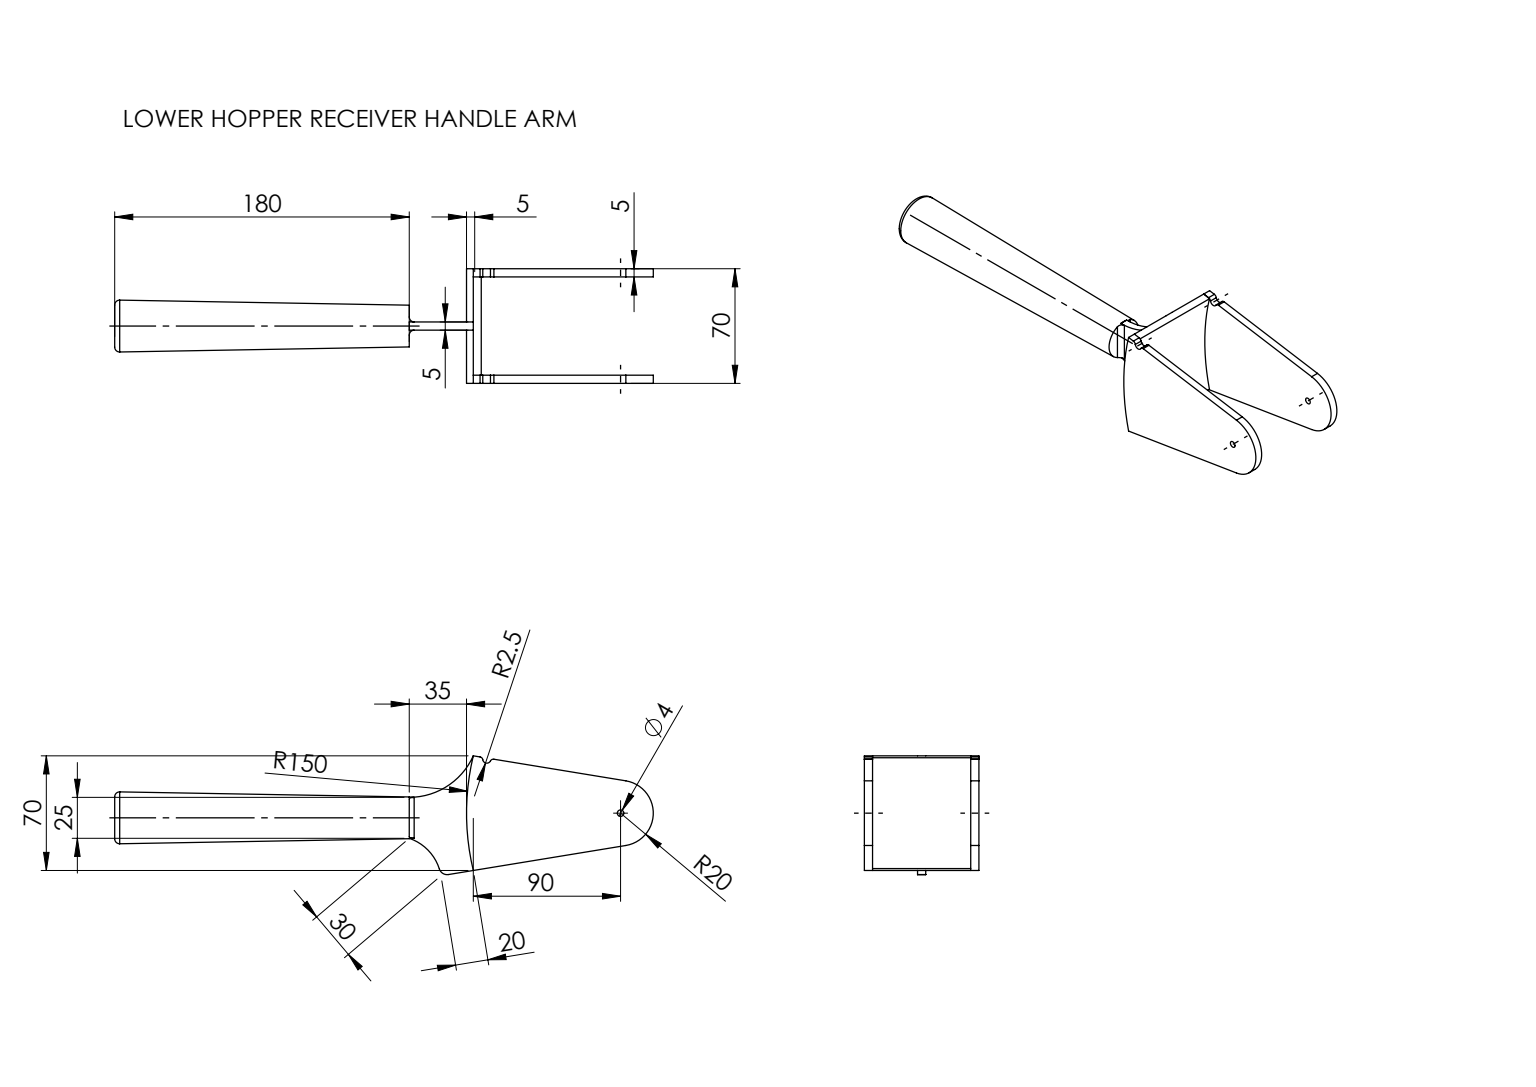
ISO-10303-21;
HEADER;
FILE_DESCRIPTION (('STEP AP214'),
    '1' );
FILE_NAME ('Lower Hopper Receiver Handle Arm.step',
    '2026-10-02T13:02:33',
    ( '' ),
    ( '' ),
    'SwSTEP 2.0',
    'SolidWorks 2026',
    '' );
FILE_SCHEMA (( 'AUTOMOTIVE_DESIGN' ));
ENDSEC;

DATA;
#29=LINE ( 'NONE', #5530, #5145 ) ;
#39=LINE ( 'NONE', #5829, #1016 ) ;
#44=VERTEX_POINT ( 'NONE', #12516 ) ;
#55=EDGE_CURVE ( 'NONE', #14250, #12234, #5712, .T. ) ;
#59=CIRCLE ( 'NONE', #13963, 20.00000000000001066 ) ;
#65=AXIS2_PLACEMENT_3D ( 'NONE', #12198, #9374, #18037 ) ;
#85=ADVANCED_FACE ( 'NONE', ( #5892 ), #18647, .T. ) ;
#86=CARTESIAN_POINT ( 'NONE',  ( -89.99999999999998579, -35.00000000000001421, 100.5765140304660861 ) ) ;
#96=CARTESIAN_POINT ( 'NONE',  ( -127.1404785156000941, 9.613695087247878135, -2.500000000000000000 ) ) ;
#99=CARTESIAN_POINT ( 'NONE',  ( -129.1404785418517918, 9.649298036820672664, 2.500000000000000000 ) ) ;
#111=CARTESIAN_POINT ( 'NONE',  ( 0.000000000000000000, 0.000000000000000000, 35.00000000000000000 ) ) ;
#116=DIRECTION ( 'NONE',  ( -0.9723968097209879646, 0.2333333333333338921, -0.000000000000000000 ) ) ;
#122=EDGE_LOOP ( 'NONE', ( #6243, #4264, #10759 ) ) ;
#125=ORIENTED_EDGE ( 'NONE', *, *, #6218, .F. ) ;
#126=CARTESIAN_POINT ( 'NONE',  ( -306.1404785418517918, -2.850701963179328668, 9.951701414186818625E-16 ) ) ;
#127=EDGE_CURVE ( 'NONE', #15127, #18093, #8457, .T. ) ;
#148=EDGE_CURVE ( 'NONE', #7107, #5722, #1632, .T. ) ;
#150=EDGE_CURVE ( 'NONE', #1792, #949, #14691, .T. ) ;
#190=CIRCLE ( 'NONE', #802, 42.89102435249441925 ) ;
#198=DIRECTION ( 'NONE',  ( 1.000000000000000000, 0.000000000000000000, -0.000000000000000000 ) ) ;
#215=EDGE_LOOP ( 'NONE', ( #10832, #6172, #11697, #10724 ) ) ;
#237=LINE ( 'NONE', #7306, #7511 ) ;
#245=CARTESIAN_POINT ( 'NONE',  ( -129.1404785418517918, 8.649298036820676217, 5.500000000000000000 ) ) ;
#246=CYLINDRICAL_SURFACE ( 'NONE', #528, 2.000000000000001776 ) ;
#266=FACE_OUTER_BOUND ( 'NONE', #3188, .T. ) ;
#273=EDGE_CURVE ( 'NONE', #17252, #3975, #18174, .T. ) ;
#286=AXIS2_PLACEMENT_3D ( 'NONE', #9882, #15657, #10154 ) ;
#290=ORIENTED_EDGE ( 'NONE', *, *, #11265, .T. ) ;
#294=VERTEX_POINT ( 'NONE', #7445 ) ;
#305=ORIENTED_EDGE ( 'NONE', *, *, #9387, .T. ) ;
#348=VECTOR ( 'NONE', #6882, 1000.000000000000000 ) ;
#381=ORIENTED_EDGE ( 'NONE', *, *, #387, .F. ) ;
#387=EDGE_CURVE ( 'NONE', #11399, #16710, #13584, .T. ) ;
#429=ORIENTED_EDGE ( 'NONE', *, *, #3774, .F. ) ;
#482=VERTEX_POINT ( 'NONE', #1195 ) ;
#514=CARTESIAN_POINT ( 'NONE',  ( -129.1404785418517918, -2.850701963179328668, 9.951701414186818625E-16 ) ) ;
#528=AXIS2_PLACEMENT_3D ( 'NONE', #2893, #8689, #14567 ) ;
#551=FILL_AREA_STYLE_COLOUR ( '', #12034 ) ;
#569=CIRCLE ( 'NONE', #2365, 150.0000000000000000 ) ;
#580=UNCERTAINTY_MEASURE_WITH_UNIT (LENGTH_MEASURE( 1.000000000000000082E-05 ), #14853, 'distance_accuracy_value', 'NONE');
#582=FACE_OUTER_BOUND ( 'NONE', #8107, .T. ) ;
#584=VERTEX_POINT ( 'NONE', #8328 ) ;
#610=VERTEX_POINT ( 'NONE', #13044 ) ;
#634=ADVANCED_FACE ( 'NONE', ( #824 ), #15404, .T. ) ;
#648=AXIS2_PLACEMENT_3D ( 'NONE', #10093, #14649, #17614 ) ;
#650=CARTESIAN_POINT ( 'NONE',  ( 55.85952145814821534, 6.938893903907228378E-15, -30.00000000000000000 ) ) ;
#651=DIRECTION ( 'NONE',  ( 0.000000000000000000, 0.000000000000000000, 1.000000000000000000 ) ) ;
#660=TOROIDAL_SURFACE ( 'NONE', #5229, 12.83663829214476060, 3.000000000000000000 ) ;
#668=EDGE_LOOP ( 'NONE', ( #10359, #125, #12635, #15355, #1976 ) ) ;
#669=EDGE_CURVE ( 'NONE', #3382, #9105, #9816, .T. ) ;
#678=CARTESIAN_POINT ( 'NONE',  ( -129.1404785418517918, -2.850701963179328668, 9.951701414186818625E-16 ) ) ;
#715=DIRECTION ( 'NONE',  ( 0.9868632313631133801, 0.1615579233078775490, 0.000000000000000000 ) ) ;
#716=DIRECTION ( 'NONE',  ( -2.735665993912342121E-16, -0.000000000000000000, -1.000000000000000000 ) ) ;
#733=EDGE_LOOP ( 'NONE', ( #1309, #17633, #9167, #16624 ) ) ;
#739=CARTESIAN_POINT ( 'NONE',  ( 3.231158466157545206, -19.73726462726228092, -35.00000000000000000 ) ) ;
#746=CARTESIAN_POINT ( 'NONE',  ( -306.0881213225399051, -2.850701963179326448, -15.83618137761393463 ) ) ;
#765=CARTESIAN_POINT ( 'NONE',  ( -128.8626752476364175, -14.87423233749613694, -4.224609204322598011 ) ) ;
#766=DIRECTION ( 'NONE',  ( -0.000000000000000000, -0.000000000000000000, -1.000000000000000000 ) ) ;
#768=CARTESIAN_POINT ( 'NONE',  ( -127.1354840320379225, 9.580137489138413898, -2.662644313562638754 ) ) ;
#769=DIRECTION ( 'NONE',  ( -0.000000000000000000, -0.000000000000000000, -1.000000000000000000 ) ) ;
#787=EDGE_CURVE ( 'NONE', #17205, #5608, #12280, .T. ) ;
#802=AXIS2_PLACEMENT_3D ( 'NONE', #11740, #14986, #10707 ) ;
#804=CARTESIAN_POINT ( 'NONE',  ( -126.1404785418517918, -15.29729532696464922, 2.500000000000000000 ) ) ;
#820=ORIENTED_EDGE ( 'NONE', *, *, #55, .F. ) ;
#822=COLOUR_RGB ( '', 0.09019608, 0.27058824, 0.51372549) ;
#824=FACE_OUTER_BOUND ( 'NONE', #12213, .T. ) ;
#846=DIRECTION ( 'NONE',  ( 0.000000000000000000, -1.000000000000000000, 0.000000000000000000 ) ) ;
#861=CARTESIAN_POINT ( 'NONE',  ( -129.1404785418517918, -15.35070196317932911, -2.500000000000000000 ) ) ;
#866=DIRECTION ( 'NONE',  ( 1.000000000000000000, -3.469446951953611033E-15, 0.000000000000000000 ) ) ;
#870=CARTESIAN_POINT ( 'NONE',  ( -77.72973689007648090, 30.96463005215034059, 30.00000000000002842 ) ) ;
#876=ORIENTED_EDGE ( 'NONE', *, *, #14228, .F. ) ;
#915=LINE ( 'NONE', #14158, #348 ) ;
#935=VECTOR ( 'NONE', #846, 1000.000000000000000 ) ;
#949=VERTEX_POINT ( 'NONE', #14168 ) ;
#970=CYLINDRICAL_SURFACE ( 'NONE', #18454, 42.89102435249441925 ) ;
#978=EDGE_CURVE ( 'NONE', #14250, #3442, #3727, .T. ) ;
#986=CARTESIAN_POINT ( 'NONE',  ( -129.1404785418517918, -2.850701963179328668, 9.951701414186818625E-16 ) ) ;
#1000=LINE ( 'NONE', #6771, #7871 ) ;
#1012=ADVANCED_FACE ( 'NONE', ( #3813 ), #9628, .F. ) ;
#1016=VECTOR ( 'NONE', #13635, 1000.000000000000000 ) ;
#1025=CYLINDRICAL_SURFACE ( 'NONE', #1765, 150.0000000000000000 ) ;
#1026=CARTESIAN_POINT ( 'NONE',  ( 0.000000000000000000, 0.000000000000000000, 35.00000000000000000 ) ) ;
#1037=ORIENTED_EDGE ( 'NONE', *, *, #6093, .T. ) ;
#1043=AXIS2_PLACEMENT_3D ( 'NONE', #16101, #1684, #10478 ) ;
#1070=CARTESIAN_POINT ( 'NONE',  ( -79.50968810220766159, 31.87664632526870889, -35.00000000000000000 ) ) ;
#1071=ADVANCED_FACE ( 'NONE', ( #5585 ), #1143, .F. ) ;
#1094=ORIENTED_EDGE ( 'NONE', *, *, #9224, .T. ) ;
#1121=CIRCLE ( 'NONE', #15923, 150.0000000000000000 ) ;
#1124=DIRECTION ( 'NONE',  ( -1.000000000000000000, 0.000000000000000000, 0.000000000000000000 ) ) ;
#1137=CARTESIAN_POINT ( 'NONE',  ( -80.37374032648909861, 30.90317544272717498, 35.00001199999999102 ) ) ;
#1143=CYLINDRICAL_SURFACE ( 'NONE', #11190, 145.0000000000000284 ) ;
#1150=B_SPLINE_CURVE_WITH_KNOTS ( 'NONE', 3,
 ( #99, #8902, #14865, #6255 ),
 .UNSPECIFIED., .F., .F.,
 ( 4, 4 ),
 ( 0.000000000000000000, 0.003000475340473869428 ),
 .UNSPECIFIED. ) ;
#1153=CARTESIAN_POINT ( 'NONE',  ( -128.4401431403265121, 9.376841461187488846, -3.563338245596201048 ) ) ;
#1161=CARTESIAN_POINT ( 'NONE',  ( -128.1404785157144204, 9.631497293019437578, -2.500000000000000000 ) ) ;
#1184=CARTESIAN_POINT ( 'NONE',  ( -90.00000000000000000, 34.99999999999999289, -2.499999999999974243 ) ) ;
#1195=CARTESIAN_POINT ( 'NONE',  ( -77.40662104346073136, 32.93835651487657401, -35.00000000000000000 ) ) ;
#1245=CARTESIAN_POINT ( 'NONE',  ( -110.7369027592740167, -34.07064978273316314, -2.500000000000000000 ) ) ;
#1247=LINE ( 'NONE', #7032, #4023 ) ;
#1255=DIRECTION ( 'NONE',  ( -2.735665993912342121E-16, -0.000000000000000000, -1.000000000000000000 ) ) ;
#1256=VECTOR ( 'NONE', #2851, 1000.000000000000000 ) ;
#1272=ORIENTED_EDGE ( 'NONE', *, *, #9509, .T. ) ;
#1274=CARTESIAN_POINT ( 'NONE',  ( -129.1404785418517918, 9.649298036820672664, 2.500000000000000000 ) ) ;
#1286=ORIENTED_EDGE ( 'NONE', *, *, #15705, .F. ) ;
#1287=DIRECTION ( 'NONE',  ( 0.000000000000000000, 0.000000000000000000, 1.000000000000000000 ) ) ;
#1309=ORIENTED_EDGE ( 'NONE', *, *, #1355, .F. ) ;
#1311=CYLINDRICAL_SURFACE ( 'NONE', #648, 2.000000000000001776 ) ;
#1312=VERTEX_POINT ( 'NONE', #13991 ) ;
#1325=EDGE_LOOP ( 'NONE', ( #11302, #17504, #9683, #6379 ) ) ;
#1341=FACE_OUTER_BOUND ( 'NONE', #6254, .T. ) ;
#1342=DIRECTION ( 'NONE',  ( 0.000000000000000000, 0.000000000000000000, 1.000000000000000000 ) ) ;
#1347=CARTESIAN_POINT ( 'NONE',  ( -90.00000000000000000, 34.99999999999999289, -30.00000000000000000 ) ) ;
#1355=EDGE_CURVE ( 'NONE', #13473, #12774, #14782, .T. ) ;
#1356=CYLINDRICAL_SURFACE ( 'NONE', #8842, 2.500000000000002220 ) ;
#1360=ORIENTED_EDGE ( 'NONE', *, *, #12905, .F. ) ;
#1363=CARTESIAN_POINT ( 'NONE',  ( -90.00000000000000000, 34.99999999999999289, -30.00000000000000000 ) ) ;
#1364=CARTESIAN_POINT ( 'NONE',  ( -126.1404785418517918, 6.938893903907228378E-15, 5.500000000000000000 ) ) ;
#1371=DIRECTION ( 'NONE',  ( 0.000000000000000000, 0.000000000000000000, 1.000000000000000000 ) ) ;
#1385=DIRECTION ( 'NONE',  ( 0.000000000000000000, 0.000000000000000000, -1.000000000000000000 ) ) ;
#1476=ORIENTED_EDGE ( 'NONE', *, *, #6473, .T. ) ;
#1483=DIRECTION ( 'NONE',  ( -0.000000000000000000, -0.000000000000000000, -1.000000000000000000 ) ) ;
#1485=AXIS2_PLACEMENT_3D ( 'NONE', #7363, #4399, #17328 ) ;
#1487=CARTESIAN_POINT ( 'NONE',  ( -126.1404785418517918, -15.29729532696464922, 2.500000000000000000 ) ) ;
#1494=EDGE_CURVE ( 'NONE', #13776, #10500, #13396, .T. ) ;
#1523=CYLINDRICAL_SURFACE ( 'NONE', #16034, 2.000000000000000000 ) ;
#1614=VERTEX_POINT ( 'NONE', #3435 ) ;
#1616=DIRECTION ( 'NONE',  ( 3.039628882124824168E-17, 0.000000000000000000, -1.000000000000000000 ) ) ;
#1623=DIRECTION ( 'NONE',  ( -1.000000000000000000, 0.000000000000000000, 0.000000000000000000 ) ) ;
#1627=ADVANCED_FACE ( 'NONE', ( #9323 ), #18078, .F. ) ;
#1628=ADVANCED_FACE ( 'NONE', ( #16839 ), #9613, .T. ) ;
#1632=LINE ( 'NONE', #7692, #9344 ) ;
#1656=CARTESIAN_POINT ( 'NONE',  ( -77.40662104346073136, 32.93835651487657401, 35.00000000000000000 ) ) ;
#1680=VERTEX_POINT ( 'NONE', #2865 ) ;
#1684=DIRECTION ( 'NONE',  ( 2.735665993912342121E-16, 0.000000000000000000, 1.000000000000000000 ) ) ;
#1685=ORIENTED_EDGE ( 'NONE', *, *, #10006, .F. ) ;
#1687=SURFACE_STYLE_USAGE ( .BOTH. , #11800 ) ;
#1707=DIRECTION ( 'NONE',  ( -0.000000000000000000, -0.000000000000000000, 1.000000000000000000 ) ) ;
#1718=ADVANCED_FACE ( 'NONE', ( #17513 ), #12778, .F. ) ;
#1726=CARTESIAN_POINT ( 'NONE',  ( -129.1404785418517918, -2.850701963179328668, 9.951701414186818625E-16 ) ) ;
#1727=VECTOR ( 'NONE', #15326, 1000.000000000000000 ) ;
#1733=EDGE_CURVE ( 'NONE', #18389, #16485, #12664, .T. ) ;
#1747=ORIENTED_EDGE ( 'NONE', *, *, #13227, .T. ) ;
#1761=EDGE_LOOP ( 'NONE', ( #6420, #11707, #14054, #2020 ) ) ;
#1765=AXIS2_PLACEMENT_3D ( 'NONE', #9732, #14062, #18386 ) ;
#1772=AXIS2_PLACEMENT_3D ( 'NONE', #111, #4368, #14237 ) ;
#1792=VERTEX_POINT ( 'NONE', #15900 ) ;
#1793=ADVANCED_FACE ( 'NONE', ( #4423 ), #6927, .F. ) ;
#1836=DIRECTION ( 'NONE',  ( -0.000000000000000000, -0.000000000000000000, -1.000000000000000000 ) ) ;
#1852=EDGE_CURVE ( 'NONE', #5489, #2351, #11341, .T. ) ;
#1857=SURFACE_SIDE_STYLE ('',( #13401 ) ) ;
#1860=FACE_OUTER_BOUND ( 'NONE', #5789, .T. ) ;
#1873=CARTESIAN_POINT ( 'NONE',  ( -129.1404785418517918, 8.649298036820674440, -5.500000000000000000 ) ) ;
#1875=DIRECTION ( 'NONE',  ( 1.000000000000000000, 0.000000000000000000, 0.000000000000000000 ) ) ;
#1876=ORIENTED_EDGE ( 'NONE', *, *, #18633, .T. ) ;
#1877=EDGE_CURVE ( 'NONE', #10500, #12364, #7467, .T. ) ;
#1900=DIRECTION ( 'NONE',  ( 1.000000000000000000, 0.000000000000000000, 0.000000000000000000 ) ) ;
#1925=DIRECTION ( 'NONE',  ( 1.000000000000000000, 0.000000000000000000, 0.000000000000000000 ) ) ;
#1942=CARTESIAN_POINT ( 'NONE',  ( 55.85952145814821534, 6.938893903907228378E-15, -2.500000000000000000 ) ) ;
#1943=CARTESIAN_POINT ( 'NONE',  ( -90.00000000000000000, 34.99999999999999289, 35.00000000000000000 ) ) ;
#1947=EDGE_CURVE ( 'NONE', #15938, #1312, #8966, .T. ) ;
#1961=CARTESIAN_POINT ( 'NONE',  ( -89.99999999999998579, -35.00000000000001421, 30.00000000000005329 ) ) ;
#1962=CYLINDRICAL_SURFACE ( 'NONE', #4186, 2.500000000000002220 ) ;
#1965=CARTESIAN_POINT ( 'NONE',  ( -90.00000000000000000, 34.99999999999999289, 35.00000000000000000 ) ) ;
#1975=EDGE_CURVE ( 'NONE', #10686, #18371, #915, .T. ) ;
#1976=ORIENTED_EDGE ( 'NONE', *, *, #16677, .F. ) ;
#1978=DIRECTION ( 'NONE',  ( 1.000000000000000000, 0.000000000000000000, 0.000000000000000000 ) ) ;
#1994=CIRCLE ( 'NONE', #13775, 150.0000000000000000 ) ;
#2011=ORIENTED_EDGE ( 'NONE', *, *, #15762, .T. ) ;
#2020=ORIENTED_EDGE ( 'NONE', *, *, #6851, .F. ) ;
#2038=DIRECTION ( 'NONE',  ( 0.000000000000000000, 0.000000000000000000, 1.000000000000000000 ) ) ;
#2054=CARTESIAN_POINT ( 'NONE',  ( -306.0881213225399051, -2.850701963179328668, 9.951701414186818625E-16 ) ) ;
#2056=AXIS2_PLACEMENT_3D ( 'NONE', #9834, #14191, #14294 ) ;
#2057=DIRECTION ( 'NONE',  ( -1.000000000000000000, 0.000000000000000000, 0.000000000000000000 ) ) ;
#2077=DIRECTION ( 'NONE',  ( 0.000000000000000000, 0.000000000000000000, -1.000000000000000000 ) ) ;
#2083=CARTESIAN_POINT ( 'NONE',  ( -90.00000000000000000, 34.99999999999999289, 35.00000000000000000 ) ) ;
#2084=DIRECTION ( 'NONE',  ( 1.000000000000000000, 0.000000000000000000, 0.000000000000000000 ) ) ;
#2105=CIRCLE ( 'NONE', #2707, 150.0000000000000000 ) ;
#2123=CARTESIAN_POINT ( 'NONE',  ( -86.18478963674542115, 32.34879426031891114, 30.00000000000002842 ) ) ;
#2133=VECTOR ( 'NONE', #18684, 1000.000000000000114 ) ;
#2146=CARTESIAN_POINT ( 'NONE',  ( 0.000000000000000000, 0.000000000000000000, 35.00000000000000000 ) ) ;
#2154=DIRECTION ( 'NONE',  ( -0.1615579233078772992, -0.9868632313631134911, 0.000000000000000000 ) ) ;
#2158=AXIS2_PLACEMENT_3D ( 'NONE', #7119, #12950, #4341 ) ;
#2176=ORIENTED_EDGE ( 'NONE', *, *, #11265, .F. ) ;
#2197=ORIENTED_EDGE ( 'NONE', *, *, #2667, .T. ) ;
#2202=DIRECTION ( 'NONE',  ( -0.000000000000000000, -0.000000000000000000, -1.000000000000000000 ) ) ;
#2208=ADVANCED_FACE ( 'NONE', ( #8277 ), #7046, .T. ) ;
#2216=ORIENTED_EDGE ( 'NONE', *, *, #5344, .F. ) ;
#2225=AXIS2_PLACEMENT_3D ( 'NONE', #3368, #16274, #10389 ) ;
#2248=CARTESIAN_POINT ( 'NONE',  ( -84.20837060243641758, 32.64545563739221024, 35.00000599999999906 ) ) ;
#2258=EDGE_LOOP ( 'NONE', ( #12744, #14922, #1094, #12317 ) ) ;
#2263=CIRCLE ( 'NONE', #18053, 2.000000000000001776 ) ;
#2264=DIRECTION ( 'NONE',  ( -1.000000000000000000, 0.000000000000000000, 0.000000000000000000 ) ) ;
#2287=AXIS2_PLACEMENT_3D ( 'NONE', #14317, #1342, #7124 ) ;
#2294=ORIENTED_EDGE ( 'NONE', *, *, #4880, .F. ) ;
#2301=CARTESIAN_POINT ( 'NONE',  ( -127.1354840320379225, -15.28154141549707035, 2.662644313562638310 ) ) ;
#2311=FACE_OUTER_BOUND ( 'NONE', #5865, .T. ) ;
#2314=DIRECTION ( 'NONE',  ( 0.000000000000000000, 1.000000000000000000, 1.224646799147353207E-16 ) ) ;
#2316=EDGE_LOOP ( 'NONE', ( #14529, #15736, #9747, #13850 ) ) ;
#2351=VERTEX_POINT ( 'NONE', #5911 ) ;
#2365=AXIS2_PLACEMENT_3D ( 'NONE', #3427, #17888, #6406 ) ;
#2371=CIRCLE ( 'NONE', #13861, 2.000000000000001776 ) ;
#2390=VERTEX_POINT ( 'NONE', #11928 ) ;
#2405=CARTESIAN_POINT ( 'NONE',  ( 55.85952145814821534, 6.938893903907228378E-15, 35.00000000000000000 ) ) ;
#2412=LINE ( 'NONE', #8380, #9979 ) ;
#2421=CARTESIAN_POINT ( 'NONE',  ( -84.20837060243641758, 32.64545563739221024, 35.00000599999999906 ) ) ;
#2449=CARTESIAN_POINT ( 'NONE',  ( -83.32982269052723723, 31.07393428812022051, 35.00001200000000523 ) ) ;
#2470=CARTESIAN_POINT ( 'NONE',  ( -126.5450966053943631, 9.599007176297428501, -2.520603730400377440 ) ) ;
#2471=DIRECTION ( 'NONE',  ( 0.000000000000000000, 0.000000000000000000, -1.000000000000000000 ) ) ;
#2477=CARTESIAN_POINT ( 'NONE',  ( -89.99999999999998579, -35.00000000000001421, 2.500000000000030198 ) ) ;
#2478=ORIENTED_EDGE ( 'NONE', *, *, #13227, .F. ) ;
#2492=AXIS2_PLACEMENT_3D ( 'NONE', #2054, #6442, #651 ) ;
#2502=EDGE_LOOP ( 'NONE', ( #15673, #8880, #4795, #16546, #6404 ) ) ;
#2514=FACE_BOUND ( 'NONE', #2700, .T. ) ;
#2531=SHAPE_REPRESENTATION_RELATIONSHIP ( 'NONE' , 'NONE' ,  #17876, #16831 ) ;
#2554=CARTESIAN_POINT ( 'NONE',  ( 55.85952145814821534, 6.938893903907228378E-15, 35.00000000000000000 ) ) ;
#2561=VERTEX_POINT ( 'NONE', #9480 ) ;
#2577=FACE_OUTER_BOUND ( 'NONE', #5940, .T. ) ;
#2578=DIRECTION ( 'NONE',  ( -0.9868632313631133801, 0.1615579233078772436, -0.000000000000000000 ) ) ;
#2606=EDGE_LOOP ( 'NONE', ( #4453, #290, #8768, #8101, #18259, #11902, #6738, #11595, #18767 ) ) ;
#2608=AXIS2_PLACEMENT_3D ( 'NONE', #4351, #18716, #16004 ) ;
#2616=VECTOR ( 'NONE', #2844, 1000.000000000000000 ) ;
#2622=DIRECTION ( 'NONE',  ( -1.000000000000000000, 0.000000000000000000, 0.000000000000000000 ) ) ;
#2624=ORIENTED_EDGE ( 'NONE', *, *, #1733, .F. ) ;
#2637=DIRECTION ( 'NONE',  ( -0.000000000000000000, -0.000000000000000000, -1.000000000000000000 ) ) ;
#2667=EDGE_CURVE ( 'NONE', #12027, #13473, #9158, .T. ) ;
#2671=DIRECTION ( 'NONE',  ( 0.000000000000000000, -1.000000000000000000, 0.000000000000000000 ) ) ;
#2674=ORIENTED_EDGE ( 'NONE', *, *, #14267, .F. ) ;
#2688=VECTOR ( 'NONE', #18062, 1000.000000000000000 ) ;
#2700=EDGE_LOOP ( 'NONE', ( #3536, #4135 ) ) ;
#2707=AXIS2_PLACEMENT_3D ( 'NONE', #1942, #12050, #17710 ) ;
#2713=CARTESIAN_POINT ( 'NONE',  ( -128.1677737538112751, 9.451028958170518024, 3.279750847804448366 ) ) ;
#2726=LINE ( 'NONE', #4126, #10310 ) ;
#2741=CARTESIAN_POINT ( 'NONE',  ( -85.86167379012967160, 34.32252072304513746, 35.00000000000000000 ) ) ;
#2775=ORIENTED_EDGE ( 'NONE', *, *, #6196, .F. ) ;
#2780=EDGE_CURVE ( 'NONE', #13776, #2561, #17653, .T. ) ;
#2842=ORIENTED_EDGE ( 'NONE', *, *, #15504, .F. ) ;
#2844=DIRECTION ( 'NONE',  ( -0.000000000000000000, -0.000000000000000000, -1.000000000000000000 ) ) ;
#2851=DIRECTION ( 'NONE',  ( -0.000000000000000000, -0.000000000000000000, -1.000000000000000000 ) ) ;
#2861=AXIS2_PLACEMENT_3D ( 'NONE', #15696, #2622, #10781 ) ;
#2865=CARTESIAN_POINT ( 'NONE',  ( -129.1404785418517918, -2.850701963179326892, -12.74754878398196389 ) ) ;
#2870=EDGE_CURVE ( 'NONE', #610, #12140, #10520, .T. ) ;
#2871=CARTESIAN_POINT ( 'NONE',  ( -129.1404785418517918, 9.649298036820672664, 2.500000000000000000 ) ) ;
#2883=CARTESIAN_POINT ( 'NONE',  ( -128.0167453206627783, 9.481696373754449070, 3.150553392547042364 ) ) ;
#2890=DIRECTION ( 'NONE',  ( 0.9868632313631133801, 0.1615579233078773547, -0.000000000000000000 ) ) ;
#2893=CARTESIAN_POINT ( 'NONE',  ( -86.18478963674542115, 32.34879426031891114, -35.00000000000000000 ) ) ;
#2895=CARTESIAN_POINT ( 'NONE',  ( -81.73462711737164454, 33.01666666666666572, -30.00000000000000355 ) ) ;
#2908=DIRECTION ( 'NONE',  ( -0.9868632313631133801, -0.1615579233078775490, 0.000000000000000000 ) ) ;
#2924=CIRCLE ( 'NONE', #15335, 29.12282187559191016 ) ;
#2941=FACE_OUTER_BOUND ( 'NONE', #733, .T. ) ;
#2951=CARTESIAN_POINT ( 'NONE',  ( -309.1404785418517918, -2.850701963179328668, 12.83663829214476237 ) ) ;
#2979=CARTESIAN_POINT ( 'NONE',  ( -84.20693962813486166, 32.64562644091790844, -35.00000000000000000 ) ) ;
#2998=EDGE_CURVE ( 'NONE', #7107, #13776, #10226, .T. ) ;
#3001=AXIS2_PLACEMENT_3D ( 'NONE', #3771, #13725, #6472 ) ;
#3023=ORIENTED_EDGE ( 'NONE', *, *, #787, .T. ) ;
#3027=ORIENTED_EDGE ( 'NONE', *, *, #1494, .F. ) ;
#3034=EDGE_LOOP ( 'NONE', ( #16222, #15224, #6139, #16013 ) ) ;
#3036=CARTESIAN_POINT ( 'NONE',  ( -129.1404785418517918, -14.35070196317933267, -5.500000000000000000 ) ) ;
#3044=DIRECTION ( 'NONE',  ( 1.000000000000000000, 0.000000000000000000, 0.000000000000000000 ) ) ;
#3046=FACE_OUTER_BOUND ( 'NONE', #2606, .T. ) ;
#3074=EDGE_LOOP ( 'NONE', ( #6524, #10962, #2478, #2775 ) ) ;
#3095=ORIENTED_EDGE ( 'NONE', *, *, #387, .T. ) ;
#3105=ADVANCED_FACE ( 'NONE', ( #16971 ), #17062, .F. ) ;
#3108=LINE ( 'NONE', #8899, #16953 ) ;
#3118=FACE_OUTER_BOUND ( 'NONE', #4884, .T. ) ;
#3160=DIRECTION ( 'NONE',  ( -0.1615579233078772992, -0.9868632313631134911, 0.000000000000000000 ) ) ;
#3163=PRESENTATION_STYLE_ASSIGNMENT (( #9236 ) ) ;
#3188=EDGE_LOOP ( 'NONE', ( #15172, #10918, #18610 ) ) ;
#3201=EDGE_CURVE ( 'NONE', #9794, #12027, #14443, .T. ) ;
#3213=MECHANICAL_DESIGN_GEOMETRIC_PRESENTATION_REPRESENTATION('',(#11387),#8064);
#3231=AXIS2_PLACEMENT_3D ( 'NONE', #15088, #4857, #16443 ) ;
#3243=ADVANCED_FACE ( 'NONE', ( #13217 ), #246, .T. ) ;
#3268=CLOSED_SHELL ( 'NONE', ( #9951, #4039, #1012, #1071, #1793, #1628, #5538, #10881, #3871, #14129, #18595, #12794, #85, #10346, #8273, #12172, #5357, #1718, #11643, #9411, #18632, #634, #13985, #3105, #4856, #13649, #18487, #1627, #18382, #14420, #13554, #13698, #12325, #5455, #11741, #8566, #11712, #11441, #2208, #7666, #18748, #3243, #13478, #7173, #7750, #17276, #15621 ) ) ;
#3272=CARTESIAN_POINT ( 'NONE',  ( -89.14047854185180597, 6.938893903907228378E-15, 100.5765140304660861 ) ) ;
#3304=CARTESIAN_POINT ( 'NONE',  ( -89.99999999999998579, -35.00000000000001421, 2.500000000000000000 ) ) ;
#3322=AXIS2_PLACEMENT_3D ( 'NONE', #7981, #15189, #10802 ) ;
#3330=CIRCLE ( 'NONE', #11804, 2.500000000000002220 ) ;
#3355=CARTESIAN_POINT ( 'NONE',  ( -86.18478963674542115, 32.34879426031891114, -30.00000000000000355 ) ) ;
#3357=AXIS2_PLACEMENT_3D ( 'NONE', #8174, #14036, #12600 ) ;
#3368=CARTESIAN_POINT ( 'NONE',  ( -90.00000000000000000, 34.99999999999999289, 100.5765140304660861 ) ) ;
#3382=VERTEX_POINT ( 'NONE', #9309 ) ;
#3389=LINE ( 'NONE', #12291, #6432 ) ;
#3391=CARTESIAN_POINT ( 'NONE',  ( -129.0554062880559343, -14.67359210495141575, -4.766626691765363688 ) ) ;
#3396=VERTEX_POINT ( 'NONE', #3424 ) ;
#3406=ORIENTED_EDGE ( 'NONE', *, *, #978, .F. ) ;
#3416=EDGE_CURVE ( 'NONE', #14596, #18395, #11106, .T. ) ;
#3420=CARTESIAN_POINT ( 'NONE',  ( -89.99999999999998579, -35.00000000000001421, 30.00000000000002487 ) ) ;
#3424=CARTESIAN_POINT ( 'NONE',  ( -79.50968810220766159, 31.87664632526870889, 30.00000000000002842 ) ) ;
#3427=CARTESIAN_POINT ( 'NONE',  ( 55.85952145814821534, 6.938893903907228378E-15, 2.500000000000000000 ) ) ;
#3435=CARTESIAN_POINT ( 'NONE',  ( -79.50968810220766159, 31.87664632526870889, -35.00000000000000000 ) ) ;
#3442=VERTEX_POINT ( 'NONE', #6944 ) ;
#3445=ORIENTED_EDGE ( 'NONE', *, *, #150, .F. ) ;
#3490=CARTESIAN_POINT ( 'NONE',  ( -309.1404785418517918, -2.850701963179326892, -12.83663829214475882 ) ) ;
#3495=ORIENTED_EDGE ( 'NONE', *, *, #10445, .T. ) ;
#3519=ORIENTED_EDGE ( 'NONE', *, *, #12303, .F. ) ;
#3536=ORIENTED_EDGE ( 'NONE', *, *, #3774, .T. ) ;
#3579=ORIENTED_EDGE ( 'NONE', *, *, #18601, .T. ) ;
#3589=VECTOR ( 'NONE', #13239, 1000.000000000000000 ) ;
#3601=CARTESIAN_POINT ( 'NONE',  ( -126.1404785418517918, 9.595891400605990995, 2.500000000000000000 ) ) ;
#3631=DIRECTION ( 'NONE',  ( 0.000000000000000000, 0.000000000000000000, 1.000000000000000000 ) ) ;
#3651=VERTEX_POINT ( 'NONE', #11668 ) ;
#3654=DIRECTION ( 'NONE',  ( 0.000000000000000000, 0.000000000000000000, 1.000000000000000000 ) ) ;
#3677=CARTESIAN_POINT ( 'NONE',  ( -126.1404785418517918, -15.29729532696464567, -2.500000000000000000 ) ) ;
#3680=CARTESIAN_POINT ( 'NONE',  ( -85.86167379012967160, 34.32252072304513746, 35.00000000000000000 ) ) ;
#3724=FACE_OUTER_BOUND ( 'NONE', #11173, .T. ) ;
#3727=LINE ( 'NONE', #9896, #11483 ) ;
#3748=VERTEX_POINT ( 'NONE', #6311 ) ;
#3762=AXIS2_PLACEMENT_3D ( 'NONE', #5266, #13869, #14273 ) ;
#3771=CARTESIAN_POINT ( 'NONE',  ( -126.1404785418517918, -2.850701963179328668, -5.500000000000000000 ) ) ;
#3774=EDGE_CURVE ( 'NONE', #12140, #610, #7877, .T. ) ;
#3799=CIRCLE ( 'NONE', #14422, 145.0000000000000284 ) ;
#3809=PLANE ( 'NONE',  #9232 ) ;
#3812=EDGE_LOOP ( 'NONE', ( #14328, #12878 ) ) ;
#3813=FACE_OUTER_BOUND ( 'NONE', #1325, .T. ) ;
#3833=CARTESIAN_POINT ( 'NONE',  ( -89.14047854185180597, 6.938893903907228378E-15, -30.00000000000000000 ) ) ;
#3839=CARTESIAN_POINT ( 'NONE',  ( -83.69844302882627574, 31.44749966561626664, 35.00001199999999812 ) ) ;
#3871=ADVANCED_FACE ( 'NONE', ( #582 ), #15062, .F. ) ;
#3880=VECTOR ( 'NONE', #18023, 1000.000000000000000 ) ;
#3891=CARTESIAN_POINT ( 'NONE',  ( -128.4401431403265121, -15.07824538754614352, 3.563338245596200160 ) ) ;
#3893=CIRCLE ( 'NONE', #18199, 12.74754878398196567 ) ;
#3919=ORIENTED_EDGE ( 'NONE', *, *, #12136, .T. ) ;
#3947=ORIENTED_EDGE ( 'NONE', *, *, #12727, .F. ) ;
#3975=VERTEX_POINT ( 'NONE', #1245 ) ;
#3976=ORIENTED_EDGE ( 'NONE', *, *, #14274, .T. ) ;
#3986=ORIENTED_EDGE ( 'NONE', *, *, #6473, .F. ) ;
#3993=ORIENTED_EDGE ( 'NONE', *, *, #6093, .F. ) ;
#4023=VECTOR ( 'NONE', #12780, 1000.000000000000000 ) ;
#4034=CARTESIAN_POINT ( 'NONE',  ( -79.50650145259169221, 31.87494681980769684, 35.00000599999999906 ) ) ;
#4039=ADVANCED_FACE ( 'NONE', ( #15092 ), #14236, .T. ) ;
#4050=CARTESIAN_POINT ( 'NONE',  ( 3.231158466157551423, 19.73726462726227737, 35.00000000000000000 ) ) ;
#4080=EDGE_LOOP ( 'NONE', ( #7014, #5618, #2294, #1360, #5467, #8933, #13419, #8424, #14819, #5962, #5132 ) ) ;
#4081=DIRECTION ( 'NONE',  ( 0.000000000000000000, 0.000000000000000000, 1.000000000000000000 ) ) ;
#4089=CIRCLE ( 'NONE', #12570, 3.000000000000000888 ) ;
#4097=CARTESIAN_POINT ( 'NONE',  ( -128.1404785157144204, -15.33290121937806205, -2.500000000000000000 ) ) ;
#4124=ORIENTED_EDGE ( 'NONE', *, *, #13537, .T. ) ;
#4126=CARTESIAN_POINT ( 'NONE',  ( 2.000000000000000000, 2.449293598294706414E-16, 35.00000000000000000 ) ) ;
#4135=ORIENTED_EDGE ( 'NONE', *, *, #2870, .T. ) ;
#4140=DIRECTION ( 'NONE',  ( -0.000000000000000000, -0.000000000000000000, -1.000000000000000000 ) ) ;
#4144=DIRECTION ( 'NONE',  ( 1.000000000000000000, 0.000000000000000000, -2.735665993912342121E-16 ) ) ;
#4149=PLANE ( 'NONE',  #2287 ) ;
#4152=CARTESIAN_POINT ( 'NONE',  ( -129.1404785418517918, 9.649298036820672664, -2.500000000000007994 ) ) ;
#4186=AXIS2_PLACEMENT_3D ( 'NONE', #11972, #10481, #13234 ) ;
#4199=PRODUCT_CONTEXT ( 'NONE', #8103, 'mechanical' ) ;
#4210=CARTESIAN_POINT ( 'NONE',  ( -85.13801595139511846, 33.83333333333333570, -30.00000000000000000 ) ) ;
#4219=CARTESIAN_POINT ( 'NONE',  ( -129.1237011781999513, 8.819295008908911271, 5.132545408516866914 ) ) ;
#4228=AXIS2_PLACEMENT_3D ( 'NONE', #514, #9143, #14913 ) ;
#4264=ORIENTED_EDGE ( 'NONE', *, *, #15989, .T. ) ;
#4278=CIRCLE ( 'NONE', #17017, 2.000000000000001776 ) ;
#4279=CARTESIAN_POINT ( 'NONE',  ( -85.86167379012967160, 34.32252072304513746, 35.00000000000000000 ) ) ;
#4283=LINE ( 'NONE', #1363, #9403 ) ;
#4288=EDGE_CURVE ( 'NONE', #294, #3396, #5891, .T. ) ;
#4341=DIRECTION ( 'NONE',  ( -1.000000000000000000, 0.000000000000000000, 0.000000000000000000 ) ) ;
#4351=CARTESIAN_POINT ( 'NONE',  ( 0.000000000000000000, 0.000000000000000000, -35.00000000000000000 ) ) ;
#4368=DIRECTION ( 'NONE',  ( -0.000000000000000000, -0.000000000000000000, -1.000000000000000000 ) ) ;
#4395=DIRECTION ( 'NONE',  ( 0.000000000000000000, 0.000000000000000000, 1.000000000000000000 ) ) ;
#4399=DIRECTION ( 'NONE',  ( -0.000000000000000000, -0.000000000000000000, -1.000000000000000000 ) ) ;
#4407=ORIENTED_EDGE ( 'NONE', *, *, #17051, .T. ) ;
#4410=CARTESIAN_POINT ( 'NONE',  ( -2.000000000000000000, 0.000000000000000000, -30.00000000000000000 ) ) ;
#4411=DIRECTION ( 'NONE',  ( 1.000000000000000000, 0.000000000000000000, -2.631994239413086031E-16 ) ) ;
#4417=CIRCLE ( 'NONE', #2608, 2.000000000000000000 ) ;
#4423=FACE_OUTER_BOUND ( 'NONE', #3034, .T. ) ;
#4434=CARTESIAN_POINT ( 'NONE',  ( -126.1404785418517918, 9.595891400605989219, -2.500000000000000000 ) ) ;
#4453=ORIENTED_EDGE ( 'NONE', *, *, #4573, .F. ) ;
#4456=ORIENTED_EDGE ( 'NONE', *, *, #14274, .F. ) ;
#4473=DIRECTION ( 'NONE',  ( -0.000000000000000000, -0.000000000000000000, -1.000000000000000000 ) ) ;
#4507=DIRECTION ( 'NONE',  ( 0.000000000000000000, 0.000000000000000000, 1.000000000000000000 ) ) ;
#4526=FACE_OUTER_BOUND ( 'NONE', #13773, .T. ) ;
#4527=DIRECTION ( 'NONE',  ( -0.000000000000000000, -0.000000000000000000, -1.000000000000000000 ) ) ;
#4540=DIRECTION ( 'NONE',  ( -0.000000000000000000, -0.000000000000000000, -1.000000000000000000 ) ) ;
#4544=DIRECTION ( 'NONE',  ( 2.735665993912342121E-16, 0.000000000000000000, 1.000000000000000000 ) ) ;
#4550=EDGE_CURVE ( 'NONE', #5489, #12882, #2105, .T. ) ;
#4551=AXIS2_PLACEMENT_3D ( 'NONE', #11371, #14616, #3044 ) ;
#4573=EDGE_CURVE ( 'NONE', #16485, #2390, #17902, .T. ) ;
#4606=EDGE_LOOP ( 'NONE', ( #381, #3495, #1272, #6713 ) ) ;
#4608=EDGE_LOOP ( 'NONE', ( #9013, #429, #18050, #7987 ) ) ;
#4617=PRESENTATION_STYLE_ASSIGNMENT (( #1687 ) ) ;
#4627=LINE ( 'NONE', #15046, #3589 ) ;
#4642=CARTESIAN_POINT ( 'NONE',  ( 0.000000000000000000, 0.000000000000000000, -30.00000000000000000 ) ) ;
#4682=DIRECTION ( 'NONE',  ( 0.000000000000000000, 0.000000000000000000, 1.000000000000000000 ) ) ;
#4697=CARTESIAN_POINT ( 'NONE',  ( -90.00000000000000000, -35.00000000000002132, 30.00000000000002842 ) ) ;
#4703=( NAMED_UNIT ( * ) SI_UNIT ( $, .STERADIAN. ) SOLID_ANGLE_UNIT ( ) );
#4720=VECTOR ( 'NONE', #17520, 1000.000000000000114 ) ;
#4729=DIRECTION ( 'NONE',  ( 3.039628882124824168E-17, 0.000000000000000000, -1.000000000000000000 ) ) ;
#4746=ORIENTED_EDGE ( 'NONE', *, *, #127, .F. ) ;
#4764=EDGE_LOOP ( 'NONE', ( #14428, #6762, #7513, #2011, #11123 ) ) ;
#4780=DIRECTION ( 'NONE',  ( 1.000000000000000000, 0.000000000000000000, -0.000000000000000000 ) ) ;
#4786=ORIENTED_EDGE ( 'NONE', *, *, #6218, .T. ) ;
#4795=ORIENTED_EDGE ( 'NONE', *, *, #12887, .T. ) ;
#4798=CARTESIAN_POINT ( 'NONE',  ( 2.000000000000000000, 2.449293598294706414E-16, -35.00000000000000000 ) ) ;
#4815=AXIS2_PLACEMENT_3D ( 'NONE', #10460, #14832, #13479 ) ;
#4856=ADVANCED_FACE ( 'NONE', ( #3046, #7415 ), #13170, .F. ) ;
#4857=DIRECTION ( 'NONE',  ( 1.000000000000000000, -0.000000000000000000, -0.000000000000000000 ) ) ;
#4863=CARTESIAN_POINT ( 'NONE',  ( -129.1404785418517918, 9.649298036820672664, -2.500000000000007994 ) ) ;
#4871=VECTOR ( 'NONE', #715, 1000.000000000000000 ) ;
#4875=DIRECTION ( 'NONE',  ( -1.000000000000000000, 0.000000000000000000, 0.000000000000000000 ) ) ;
#4880=EDGE_CURVE ( 'NONE', #584, #18389, #7398, .T. ) ;
#4884=EDGE_LOOP ( 'NONE', ( #9777, #6067, #17131, #820 ) ) ;
#4887=ORIENTED_EDGE ( 'NONE', *, *, #5076, .T. ) ;
#4938=ORIENTED_EDGE ( 'NONE', *, *, #1494, .T. ) ;
#4948=EDGE_CURVE ( 'NONE', #6209, #16318, #3108, .T. ) ;
#4955=PLANE ( 'NONE',  #5770 ) ;
#4969=EDGE_CURVE ( 'NONE', #2351, #3651, #4627, .T. ) ;
#4980=AXIS2_PLACEMENT_3D ( 'NONE', #9810, #2314, #15579 ) ;
#5002=DIRECTION ( 'NONE',  ( -0.000000000000000000, -0.000000000000000000, -1.000000000000000000 ) ) ;
#5068=AXIS2_PLACEMENT_3D ( 'NONE', #3304, #13638, #10513 ) ;
#5072=DIRECTION ( 'NONE',  ( -0.000000000000000000, -0.000000000000000000, -1.000000000000000000 ) ) ;
#5076=EDGE_CURVE ( 'NONE', #5608, #14700, #12187, .T. ) ;
#5087=( GEOMETRIC_REPRESENTATION_CONTEXT ( 3 ) GLOBAL_UNCERTAINTY_ASSIGNED_CONTEXT ( ( #580 ) ) GLOBAL_UNIT_ASSIGNED_CONTEXT ( ( #14853, #15036, #17648 ) ) REPRESENTATION_CONTEXT ( 'NONE', 'WORKASPACE' ) );
#5094=VECTOR ( 'NONE', #9866, 1000.000000000000000 ) ;
#5118=VECTOR ( 'NONE', #16253, 1000.000000000000114 ) ;
#5130=AXIS2_PLACEMENT_3D ( 'NONE', #8094, #16749, #5450 ) ;
#5132=ORIENTED_EDGE ( 'NONE', *, *, #12297, .T. ) ;
#5139=AXIS2_PLACEMENT_3D ( 'NONE', #15398, #15435, #18520 ) ;
#5145=VECTOR ( 'NONE', #2578, 1000.000000000000114 ) ;
#5154=CARTESIAN_POINT ( 'NONE',  ( -127.5060788346647200, -15.25314381392001728, 2.821239268406352974 ) ) ;
#5179=CIRCLE ( 'NONE', #10016, 20.00000000000001066 ) ;
#5212=CARTESIAN_POINT ( 'NONE',  ( -129.0020721423141481, 9.044883704321415863, -4.579216830445306030 ) ) ;
#5213=ORIENTED_EDGE ( 'NONE', *, *, #1947, .T. ) ;
#5221=CYLINDRICAL_SURFACE ( 'NONE', #15011, 150.0000000000000000 ) ;
#5229=AXIS2_PLACEMENT_3D ( 'NONE', #126, #14147, #4081 ) ;
#5254=CARTESIAN_POINT ( 'NONE',  ( -128.1659926135409933, -15.15280585534915225, 3.278196957010496959 ) ) ;
#5257=CARTESIAN_POINT ( 'NONE',  ( -138.4775067298212718, -42.93618108924343346, 2.500000000000000000 ) ) ;
#5262=DIRECTION ( 'NONE',  ( 0.000000000000000000, 0.000000000000000000, 1.000000000000000000 ) ) ;
#5266=CARTESIAN_POINT ( 'NONE',  ( -105.9742111339482307, -32.54855632894931716, 2.500000000000000000 ) ) ;
#5274=EDGE_CURVE ( 'NONE', #16906, #18093, #14225, .T. ) ;
#5279=DIRECTION ( 'NONE',  ( 1.000000000000000000, 0.000000000000000000, 0.000000000000000000 ) ) ;
#5311=CARTESIAN_POINT ( 'NONE',  ( -126.9394941819792280, 9.589416411885151703, -2.601363783521511763 ) ) ;
#5314=ORIENTED_EDGE ( 'NONE', *, *, #55, .T. ) ;
#5335=ORIENTED_EDGE ( 'NONE', *, *, #7026, .F. ) ;
#5344=EDGE_CURVE ( 'NONE', #14700, #18093, #6409, .T. ) ;
#5345=EDGE_CURVE ( 'NONE', #12027, #18395, #6941, .T. ) ;
#5349=CARTESIAN_POINT ( 'NONE',  ( -128.5628356445764098, -15.03429919720559482, 3.719291248522907711 ) ) ;
#5355=VECTOR ( 'NONE', #5879, 1000.000000000000000 ) ;
#5357=ADVANCED_FACE ( 'NONE', ( #8714 ), #1523, .F. ) ;
#5364=DIRECTION ( 'NONE',  ( 1.000000000000000000, 0.000000000000000000, -3.469446951953612217E-16 ) ) ;
#5378=DIRECTION ( 'NONE',  ( 1.000000000000000000, 0.000000000000000000, 0.000000000000000000 ) ) ;
#5386=CARTESIAN_POINT ( 'NONE',  ( -82.39751269876940398, 30.59191086097347778, 35.00001199999999812 ) ) ;
#5415=AXIS2_PLACEMENT_3D ( 'NONE', #12498, #6744, #15345 ) ;
#5426=VECTOR ( 'NONE', #14407, 1000.000000000000227 ) ;
#5450=DIRECTION ( 'NONE',  ( -1.000000000000000000, -6.938893903907222067E-15, 0.000000000000000000 ) ) ;
#5455=ADVANCED_FACE ( 'NONE', ( #266 ), #6509, .F. ) ;
#5467=ORIENTED_EDGE ( 'NONE', *, *, #9509, .F. ) ;
#5489=VERTEX_POINT ( 'NONE', #5552 ) ;
#5501=CARTESIAN_POINT ( 'NONE',  ( -128.7747222983995528, 9.230544287383699142, -4.051035741711870308 ) ) ;
#5507=DIRECTION ( 'NONE',  ( -0.000000000000000000, -0.000000000000000000, -1.000000000000000000 ) ) ;
#5530=CARTESIAN_POINT ( 'NONE',  ( -90.00000000000000000, 34.99999999999999289, 35.00000000000000000 ) ) ;
#5537=LINE ( 'NONE', #5729, #17015 ) ;
#5538=ADVANCED_FACE ( 'NONE', ( #15578 ), #1025, .T. ) ;
#5552=CARTESIAN_POINT ( 'NONE',  ( -89.99999999999998579, -35.00000000000001421, -2.499999999999974243 ) ) ;
#5566=LINE ( 'NONE', #11315, #2133 ) ;
#5569=CARTESIAN_POINT ( 'NONE',  ( -127.5081579206796221, 9.551524140464916712, 2.822349119005437501 ) ) ;
#5580=CARTESIAN_POINT ( 'NONE',  ( -79.78608161301387725, 31.42857711355109274, 35.00001200000000523 ) ) ;
#5585=FACE_OUTER_BOUND ( 'NONE', #4606, .T. ) ;
#5608=VERTEX_POINT ( 'NONE', #8939 ) ;
#5612=AXIS2_PLACEMENT_3D ( 'NONE', #1026, #15500, #12539 ) ;
#5616=DIRECTION ( 'NONE',  ( -0.000000000000000000, -0.000000000000000000, -1.000000000000000000 ) ) ;
#5618=ORIENTED_EDGE ( 'NONE', *, *, #14968, .T. ) ;
#5620=EDGE_CURVE ( 'NONE', #10500, #17370, #6303, .T. ) ;
#5624=DIRECTION ( 'NONE',  ( -0.9868632313631133801, 0.1615579233078772714, 2.699728182682517290E-16 ) ) ;
#5638=ORIENTED_EDGE ( 'NONE', *, *, #18601, .F. ) ;
#5670=EDGE_LOOP ( 'NONE', ( #9242, #10762, #3445, #9129, #3947, #6361, #7881, #3095, #8995, #9799, #5728 ) ) ;
#5694=DIRECTION ( 'NONE',  ( -1.000000000000000000, 0.000000000000000000, 0.000000000000000000 ) ) ;
#5712=LINE ( 'NONE', #4279, #5094 ) ;
#5722=VERTEX_POINT ( 'NONE', #18561 ) ;
#5728=ORIENTED_EDGE ( 'NONE', *, *, #7403, .T. ) ;
#5729=CARTESIAN_POINT ( 'NONE',  ( -110.7369027592740167, -34.07064978273316314, 2.500000000000000000 ) ) ;
#5755=AXIS2_PLACEMENT_3D ( 'NONE', #1943, #3160, #17711 ) ;
#5756=AXIS2_PLACEMENT_3D ( 'NONE', #10829, #16652, #3631 ) ;
#5764=CARTESIAN_POINT ( 'NONE',  ( -128.5664531142841440, 9.331354376930727668, 3.724467847532855647 ) ) ;
#5765=AXIS2_PLACEMENT_3D ( 'NONE', #10444, #1836, #1925 ) ;
#5770=AXIS2_PLACEMENT_3D ( 'NONE', #7649, #13482, #4780 ) ;
#5775=CARTESIAN_POINT ( 'NONE',  ( -77.72973689007648090, 30.96463005215034059, -35.00000000000000000 ) ) ;
#5779=ORIENTED_EDGE ( 'NONE', *, *, #8584, .T. ) ;
#5789=EDGE_LOOP ( 'NONE', ( #13960, #12487, #4887, #18586, #14410, #6827, #5997, #12112, #14473 ) ) ;
#5794=CARTESIAN_POINT ( 'NONE',  ( -2.000000000000000000, 0.000000000000000000, 35.00000000000000000 ) ) ;
#5801=ORIENTED_EDGE ( 'NONE', *, *, #12727, .T. ) ;
#5829=CARTESIAN_POINT ( 'NONE',  ( -90.00000000000001421, 34.99999999999996447, 2.500000000000000000 ) ) ;
#5858=CARTESIAN_POINT ( 'NONE',  ( -79.50968810220766159, 31.87664632526870889, -30.00000000000000355 ) ) ;
#5865=EDGE_LOOP ( 'NONE', ( #11447, #12404 ) ) ;
#5872=VERTEX_POINT ( 'NONE', #9791 ) ;
#5874=PLANE ( 'NONE',  #15066 ) ;
#5876=FACE_OUTER_BOUND ( 'NONE', #2258, .T. ) ;
#5879=DIRECTION ( 'NONE',  ( 0.9868632313631133801, 0.1615579233078775490, 0.000000000000000000 ) ) ;
#5891=LINE ( 'NONE', #14607, #11495 ) ;
#5892=FACE_OUTER_BOUND ( 'NONE', #9347, .T. ) ;
#5894=VERTEX_POINT ( 'NONE', #739 ) ;
#5910=ORIENTED_EDGE ( 'NONE', *, *, #150, .T. ) ;
#5911=CARTESIAN_POINT ( 'NONE',  ( -89.99999999999998579, -35.00000000000001421, -30.00000000000000355 ) ) ;
#5937=ORIENTED_EDGE ( 'NONE', *, *, #15974, .F. ) ;
#5939=CIRCLE ( 'NONE', #8949, 12.83663829214476060 ) ;
#5940=EDGE_LOOP ( 'NONE', ( #3406, #5314, #4407, #10524 ) ) ;
#5962=ORIENTED_EDGE ( 'NONE', *, *, #1947, .F. ) ;
#5963=LINE ( 'NONE', #13243, #9288 ) ;
#5972=CARTESIAN_POINT ( 'NONE',  ( -86.18478963674542115, 32.34879426031891114, -35.00000000000000000 ) ) ;
#5997=ORIENTED_EDGE ( 'NONE', *, *, #4550, .F. ) ;
#6032=CYLINDRICAL_SURFACE ( 'NONE', #10731, 2.000000000000001776 ) ;
#6047=DIRECTION ( 'NONE',  ( -1.000000000000000000, 0.000000000000000000, 0.000000000000000000 ) ) ;
#6058=EDGE_CURVE ( 'NONE', #1680, #17205, #17142, .T. ) ;
#6067=ORIENTED_EDGE ( 'NONE', *, *, #4948, .F. ) ;
#6074=CARTESIAN_POINT ( 'NONE',  ( 0.000000000000000000, 0.000000000000000000, 30.00000000000000000 ) ) ;
#6093=EDGE_CURVE ( 'NONE', #14700, #9368, #9933, .T. ) ;
#6111=CARTESIAN_POINT ( 'NONE',  ( -90.00000000000000000, 34.99999999999999289, 35.00000000000000000 ) ) ;
#6120=CARTESIAN_POINT ( 'NONE',  ( -129.1404785418517918, -15.35070196317932911, 2.500000000000000000 ) ) ;
#6139=ORIENTED_EDGE ( 'NONE', *, *, #9387, .F. ) ;
#6140=ORIENTED_EDGE ( 'NONE', *, *, #18633, .F. ) ;
#6144=ORIENTED_EDGE ( 'NONE', *, *, #18375, .F. ) ;
#6155=CARTESIAN_POINT ( 'NONE',  ( 3.231158466157545206, -19.73726462726228092, -30.00000000000000000 ) ) ;
#6156=( NAMED_UNIT ( * ) PLANE_ANGLE_UNIT ( ) SI_UNIT ( $, .RADIAN. ) );
#6172=ORIENTED_EDGE ( 'NONE', *, *, #1975, .T. ) ;
#6181=CARTESIAN_POINT ( 'NONE',  ( 55.85952145814821534, 6.938893903907228378E-15, 2.500000000000000000 ) ) ;
#6196=EDGE_CURVE ( 'NONE', #18395, #7533, #4089, .T. ) ;
#6209=VERTEX_POINT ( 'NONE', #17495 ) ;
#6218=EDGE_CURVE ( 'NONE', #3442, #7107, #1994, .T. ) ;
#6243=ORIENTED_EDGE ( 'NONE', *, *, #6533, .F. ) ;
#6254=EDGE_LOOP ( 'NONE', ( #11787, #16718 ) ) ;
#6255=CARTESIAN_POINT ( 'NONE',  ( -126.1404785418517918, 9.595891400605990995, 2.500000000000000000 ) ) ;
#6261=ORIENTED_EDGE ( 'NONE', *, *, #2780, .F. ) ;
#6270=CARTESIAN_POINT ( 'NONE',  ( -128.4427290061107101, -15.07742888475873677, -3.566331213966875691 ) ) ;
#6290=AXIS2_PLACEMENT_3D ( 'NONE', #8781, #11686, #4507 ) ;
#6303=LINE ( 'NONE', #15191, #2688 ) ;
#6311=CARTESIAN_POINT ( 'NONE',  ( -85.13801595139509004, -33.83333333333328596, -30.00000000000000000 ) ) ;
#6361=ORIENTED_EDGE ( 'NONE', *, *, #1877, .T. ) ;
#6379=ORIENTED_EDGE ( 'NONE', *, *, #11615, .F. ) ;
#6404=ORIENTED_EDGE ( 'NONE', *, *, #1852, .F. ) ;
#6406=DIRECTION ( 'NONE',  ( 1.000000000000000000, 0.000000000000000000, 0.000000000000000000 ) ) ;
#6409=B_SPLINE_CURVE_WITH_KNOTS ( 'NONE', 3,
 ( #4434, #96, #1161, #4152 ),
 .UNSPECIFIED., .F., .F.,
 ( 4, 4 ),
 ( 0.000000000000000000, 0.003000475340473870295 ),
 .UNSPECIFIED. ) ;
#6418=PLANE ( 'NONE',  #5755 ) ;
#6420=ORIENTED_EDGE ( 'NONE', *, *, #16102, .F. ) ;
#6432=VECTOR ( 'NONE', #13714, 1000.000000000000000 ) ;
#6441=DIRECTION ( 'NONE',  ( -0.000000000000000000, -0.000000000000000000, -1.000000000000000000 ) ) ;
#6442=DIRECTION ( 'NONE',  ( 1.000000000000000000, -0.000000000000000000, -0.000000000000000000 ) ) ;
#6472=DIRECTION ( 'NONE',  ( 0.000000000000000000, 0.000000000000000000, 1.000000000000000000 ) ) ;
#6473=EDGE_CURVE ( 'NONE', #17580, #15127, #190, .T. ) ;
#6474=ORIENTED_EDGE ( 'NONE', *, *, #9956, .F. ) ;
#6490=EDGE_LOOP ( 'NONE', ( #9178, #10360 ) ) ;
#6497=DIRECTION ( 'NONE',  ( 1.000000000000000000, -3.469446951953611033E-15, 0.000000000000000000 ) ) ;
#6509=PLANE ( 'NONE',  #5756 ) ;
#6524=ORIENTED_EDGE ( 'NONE', *, *, #3416, .F. ) ;
#6533=EDGE_CURVE ( 'NONE', #9368, #1680, #11667, .T. ) ;
#6540=DIRECTION ( 'NONE',  ( -1.000000000000000000, 0.000000000000000000, 0.000000000000000000 ) ) ;
#6544=CARTESIAN_POINT ( 'NONE',  ( -129.0548615328497704, 8.973171863034172802, -4.764204982952881196 ) ) ;
#6559=CIRCLE ( 'NONE', #17150, 20.00000000000001066 ) ;
#6561=ORIENTED_EDGE ( 'NONE', *, *, #15989, .F. ) ;
#6579=ORIENTED_EDGE ( 'NONE', *, *, #14835, .F. ) ;
#6586=CARTESIAN_POINT ( 'NONE',  ( -129.0020721423141197, -14.74628763068006876, 4.579216830445306030 ) ) ;
#6628=CIRCLE ( 'NONE', #15992, 2.000000000000001776 ) ;
#6644=EDGE_CURVE ( 'NONE', #16906, #584, #12510, .T. ) ;
#6692=CARTESIAN_POINT ( 'NONE',  ( -129.1404785418517918, -14.35070196317933444, 5.500000000000000000 ) ) ;
#6699=CARTESIAN_POINT ( 'NONE',  ( -85.13801595139509004, -33.83333333333328596, 29.99999999999997158 ) ) ;
#6706=EDGE_LOOP ( 'NONE', ( #11537, #8793, #17565, #15143, #11711, #8332 ) ) ;
#6712=DIRECTION ( 'NONE',  ( -0.000000000000000000, -0.000000000000000000, -1.000000000000000000 ) ) ;
#6713=ORIENTED_EDGE ( 'NONE', *, *, #9464, .F. ) ;
#6738=ORIENTED_EDGE ( 'NONE', *, *, #9657, .F. ) ;
#6744=DIRECTION ( 'NONE',  ( -1.000000000000000000, 0.000000000000000000, 0.000000000000000000 ) ) ;
#6745=DIRECTION ( 'NONE',  ( 1.000000000000000000, -3.469446951953611033E-15, 0.000000000000000000 ) ) ;
#6762=ORIENTED_EDGE ( 'NONE', *, *, #15332, .T. ) ;
#6771=CARTESIAN_POINT ( 'NONE',  ( -89.99999999999998579, -35.00000000000001421, 2.500000000000000000 ) ) ;
#6800=EDGE_LOOP ( 'NONE', ( #16950, #8358, #3919, #2842 ) ) ;
#6809=ORIENTED_EDGE ( 'NONE', *, *, #5345, .T. ) ;
#6817=CARTESIAN_POINT ( 'NONE',  ( 0.000000000000000000, 0.000000000000000000, 35.00000000000000000 ) ) ;
#6827=ORIENTED_EDGE ( 'NONE', *, *, #15332, .F. ) ;
#6837=CARTESIAN_POINT ( 'NONE',  ( -128.0119535342735162, 9.482588595290904365, -3.146712427857100813 ) ) ;
#6843=EDGE_CURVE ( 'NONE', #15127, #18093, #17788, .T. ) ;
#6851=EDGE_CURVE ( 'NONE', #9656, #13932, #13209, .T. ) ;
#6882=DIRECTION ( 'NONE',  ( -0.000000000000000000, -0.000000000000000000, 1.000000000000000000 ) ) ;
#6908=EDGE_CURVE ( 'NONE', #10401, #2351, #9091, .T. ) ;
#6918=LINE ( 'NONE', #8236, #935 ) ;
#6924=CIRCLE ( 'NONE', #12948, 5.000000000000004441 ) ;
#6927=CYLINDRICAL_SURFACE ( 'NONE', #2158, 2.000000000000000000 ) ;
#6939=( GEOMETRIC_REPRESENTATION_CONTEXT ( 3 ) GLOBAL_UNCERTAINTY_ASSIGNED_CONTEXT ( ( #18038 ) ) GLOBAL_UNIT_ASSIGNED_CONTEXT ( ( #13334, #6156, #4703 ) ) REPRESENTATION_CONTEXT ( 'NONE', 'WORKASPACE' ) );
#6941=LINE ( 'NONE', #15910, #8162 ) ;
#6944=CARTESIAN_POINT ( 'NONE',  ( -90.00000000000000000, 34.99999999999999289, 35.00000000000000000 ) ) ;
#6978=AXIS2_PLACEMENT_3D ( 'NONE', #10780, #5002, #16596 ) ;
#7002=LINE ( 'NONE', #8396, #16381 ) ;
#7008=CARTESIAN_POINT ( 'NONE',  ( -129.1404785418517918, 8.737252551174764292, 5.316095106350545940 ) ) ;
#7009=CARTESIAN_POINT ( 'NONE',  ( -105.1664215174088213, -37.48287248576487940, 2.500000000000000000 ) ) ;
#7014=ORIENTED_EDGE ( 'NONE', *, *, #16058, .T. ) ;
#7026=EDGE_CURVE ( 'NONE', #9621, #17252, #7002, .T. ) ;
#7032=CARTESIAN_POINT ( 'NONE',  ( -94.14047854185179176, 6.938893903907228378E-15, 35.00000000000000000 ) ) ;
#7041=DIRECTION ( 'NONE',  ( -1.000000000000000000, 0.000000000000000000, 0.000000000000000000 ) ) ;
#7045=ORIENTED_EDGE ( 'NONE', *, *, #14267, .T. ) ;
#7046=TOROIDAL_SURFACE ( 'NONE', #3357, 12.83663829214476060, 3.000000000000000000 ) ;
#7069=ORIENTED_EDGE ( 'NONE', *, *, #13853, .F. ) ;
#7077=VECTOR ( 'NONE', #17840, 1000.000000000000227 ) ;
#7107=VERTEX_POINT ( 'NONE', #8679 ) ;
#7119=CARTESIAN_POINT ( 'NONE',  ( 0.000000000000000000, 0.000000000000000000, 35.00000000000000000 ) ) ;
#7122=CARTESIAN_POINT ( 'NONE',  ( -89.99999999999998579, -35.00000000000001421, 35.00000000000000000 ) ) ;
#7124=DIRECTION ( 'NONE',  ( 1.000000000000000000, 0.000000000000000000, -0.000000000000000000 ) ) ;
#7170=ORIENTED_EDGE ( 'NONE', *, *, #148, .T. ) ;
#7173=ADVANCED_FACE ( 'NONE', ( #17507 ), #1311, .T. ) ;
#7259=SHAPE_DEFINITION_REPRESENTATION ( #16674, #17876 ) ;
#7275=CARTESIAN_POINT ( 'NONE',  ( -127.1404785156000941, -15.31509901360653636, 2.500000000000000000 ) ) ;
#7277=EDGE_CURVE ( 'NONE', #13253, #3382, #13507, .T. ) ;
#7306=CARTESIAN_POINT ( 'NONE',  ( 3.231158466157545206, -19.73726462726228092, 35.00000000000000000 ) ) ;
#7319=CARTESIAN_POINT ( 'NONE',  ( -90.00000000000001421, 34.99999999999996447, 2.500000000000000000 ) ) ;
#7339=CARTESIAN_POINT ( 'NONE',  ( -90.00000000000000000, 34.99999999999999289, 100.5765140304660861 ) ) ;
#7363=CARTESIAN_POINT ( 'NONE',  ( -138.4775067298212718, -42.93618108924343346, 2.500000000000000000 ) ) ;
#7364=CARTESIAN_POINT ( 'NONE',  ( -90.00000000000000000, 34.99999999999999289, -35.00000000000000000 ) ) ;
#7391=CARTESIAN_POINT ( 'NONE',  ( -94.14047854185177755, -35.00000000000001421, 30.00000000000002487 ) ) ;
#7395=DIRECTION ( 'NONE',  ( 1.000000000000000000, 0.000000000000000000, 0.000000000000000000 ) ) ;
#7396=DIRECTION ( 'NONE',  ( -1.000000000000000000, 0.000000000000000000, 0.000000000000000000 ) ) ;
#7398=LINE ( 'NONE', #1347, #5426 ) ;
#7403=EDGE_CURVE ( 'NONE', #12234, #6209, #4278, .T. ) ;
#7410=CIRCLE ( 'NONE', #2861, 12.83663829214476060 ) ;
#7415=FACE_BOUND ( 'NONE', #6490, .T. ) ;
#7441=EDGE_CURVE ( 'NONE', #13253, #9794, #11276, .T. ) ;
#7445=CARTESIAN_POINT ( 'NONE',  ( -79.50650145259169221, 31.87494681980769684, 35.00000599999999906 ) ) ;
#7453=CARTESIAN_POINT ( 'NONE',  ( -129.1404785418517918, -2.850701963179328668, 12.74754878398196745 ) ) ;
#7460=VECTOR ( 'NONE', #2471, 1000.000000000000000 ) ;
#7465=FACE_OUTER_BOUND ( 'NONE', #4764, .T. ) ;
#7467=LINE ( 'NONE', #4697, #10323 ) ;
#7473=DIRECTION ( 'NONE',  ( 0.000000000000000000, 0.000000000000000000, 1.000000000000000000 ) ) ;
#7485=CIRCLE ( 'NONE', #10479, 2.000000000000001776 ) ;
#7490=CARTESIAN_POINT ( 'NONE',  ( -89.99999999999998579, -35.00000000000001421, -30.00000000000000000 ) ) ;
#7494=EDGE_LOOP ( 'NONE', ( #15982, #16200, #11665, #17114 ) ) ;
#7501=ORIENTED_EDGE ( 'NONE', *, *, #6058, .T. ) ;
#7511=VECTOR ( 'NONE', #11618, 1000.000000000000000 ) ;
#7513=ORIENTED_EDGE ( 'NONE', *, *, #6644, .T. ) ;
#7533=VERTEX_POINT ( 'NONE', #2951 ) ;
#7539=CARTESIAN_POINT ( 'NONE',  ( -89.99999999999998579, -35.00000000000001421, 35.00000000000000000 ) ) ;
#7546=CARTESIAN_POINT ( 'NONE',  ( -85.86167379012967160, 34.32252072304513746, 30.00000000000002487 ) ) ;
#7562=AXIS2_PLACEMENT_3D ( 'NONE', #13989, #12173, #5279 ) ;
#7577=DIRECTION ( 'NONE',  ( -0.000000000000000000, -0.000000000000000000, 1.000000000000000000 ) ) ;
#7628=DIRECTION ( 'NONE',  ( -0.1615579233078772992, -0.9868632313631134911, 0.000000000000000000 ) ) ;
#7649=CARTESIAN_POINT ( 'NONE',  ( 55.85952145814821534, 6.938893903907228378E-15, 35.00000000000000000 ) ) ;
#7650=( LENGTH_UNIT ( ) NAMED_UNIT ( * ) SI_UNIT ( .MILLI., .METRE. ) );
#7666=ADVANCED_FACE ( 'NONE', ( #9950 ), #1356, .F. ) ;
#7670=FACE_OUTER_BOUND ( 'NONE', #7494, .T. ) ;
#7680=ORIENTED_EDGE ( 'NONE', *, *, #2780, .T. ) ;
#7690=AXIS2_PLACEMENT_3D ( 'NONE', #650, #6441, #5378 ) ;
#7692=CARTESIAN_POINT ( 'NONE',  ( -94.14047854185179176, 6.938893903907228378E-15, 35.00000000000000000 ) ) ;
#7731=( NAMED_UNIT ( * ) PLANE_ANGLE_UNIT ( ) SI_UNIT ( $, .RADIAN. ) );
#7747=DIRECTION ( 'NONE',  ( -0.000000000000000000, -0.000000000000000000, -1.000000000000000000 ) ) ;
#7750=ADVANCED_FACE ( 'NONE', ( #3118 ), #9094, .T. ) ;
#7827=DIRECTION ( 'NONE',  ( 1.000000000000000000, 0.000000000000000000, -0.000000000000000000 ) ) ;
#7833=VECTOR ( 'NONE', #8625, 1000.000000000000000 ) ;
#7844=DIRECTION ( 'NONE',  ( -0.9868632313631133801, -0.1615579233078775490, 0.000000000000000000 ) ) ;
#7848=DIRECTION ( 'NONE',  ( -1.000000000000000000, 0.000000000000000000, 0.000000000000000000 ) ) ;
#7868=EDGE_CURVE ( 'NONE', #1312, #10401, #59, .T. ) ;
#7871=VECTOR ( 'NONE', #2202, 1000.000000000000000 ) ;
#7877=CIRCLE ( 'NONE', #10887, 2.000000000000000000 ) ;
#7881=ORIENTED_EDGE ( 'NONE', *, *, #14833, .T. ) ;
#7921=FACE_OUTER_BOUND ( 'NONE', #9971, .T. ) ;
#7942=CARTESIAN_POINT ( 'NONE',  ( -89.99999999999998579, -35.00000000000001421, 35.00000000000000000 ) ) ;
#7973=DIRECTION ( 'NONE',  ( -1.000000000000000000, 0.000000000000000000, 0.000000000000000000 ) ) ;
#7981=CARTESIAN_POINT ( 'NONE',  ( -90.00000000000000000, 34.99999999999999289, 35.00000000000000000 ) ) ;
#7987=ORIENTED_EDGE ( 'NONE', *, *, #14331, .F. ) ;
#8006=CARTESIAN_POINT ( 'NONE',  ( -77.72973689007648090, 30.96463005215034059, 35.00000000000000000 ) ) ;
#8012=PRODUCT_DEFINITION ( 'UNKNOWN', '', #18746, #14969 ) ;
#8027=CARTESIAN_POINT ( 'NONE',  ( -81.61394393281571524, 30.50583143108602613, 35.00001199999999812 ) ) ;
#8064=( GEOMETRIC_REPRESENTATION_CONTEXT ( 3 ) GLOBAL_UNCERTAINTY_ASSIGNED_CONTEXT ( ( #9101 ) ) GLOBAL_UNIT_ASSIGNED_CONTEXT ( ( #7650, #7731, #8955 ) ) REPRESENTATION_CONTEXT ( 'NONE', 'WORKASPACE' ) );
#8094=CARTESIAN_POINT ( 'NONE',  ( -77.72973689007648090, 30.96463005215034059, -30.00000000000000355 ) ) ;
#8099=CARTESIAN_POINT ( 'NONE',  ( -94.14047854185179176, -35.00000000000001421, -30.00000000000000355 ) ) ;
#8101=ORIENTED_EDGE ( 'NONE', *, *, #11264, .T. ) ;
#8103=APPLICATION_CONTEXT ( 'automotive_design' ) ;
#8107=EDGE_LOOP ( 'NONE', ( #16809, #10960, #5213, #10347 ) ) ;
#8108=EDGE_LOOP ( 'NONE', ( #13930, #11217, #10573, #1876, #5779, #12069, #15785, #1476, #17897 ) ) ;
#8129=CIRCLE ( 'NONE', #16606, 145.0000000000000284 ) ;
#8131=CARTESIAN_POINT ( 'NONE',  ( -84.08787250788334688, 32.13287136044273495, 35.00001199999999812 ) ) ;
#8139=VECTOR ( 'NONE', #8827, 1000.000000000000227 ) ;
#8147=CARTESIAN_POINT ( 'NONE',  ( 0.000000000000000000, 0.000000000000000000, -35.00000000000000000 ) ) ;
#8161=DIRECTION ( 'NONE',  ( 0.000000000000000000, 0.000000000000000000, 1.000000000000000000 ) ) ;
#8162=VECTOR ( 'NONE', #12677, 1000.000000000000114 ) ;
#8165=EDGE_LOOP ( 'NONE', ( #14904, #16483, #14594, #15128, #6474, #8178 ) ) ;
#8169=CIRCLE ( 'NONE', #5765, 150.0000000000000000 ) ;
#8171=AXIS2_PLACEMENT_3D ( 'NONE', #13866, #11212, #5262 ) ;
#8174=CARTESIAN_POINT ( 'NONE',  ( -306.1404785418517918, -2.850701963179328668, 9.951701414186818625E-16 ) ) ;
#8178=ORIENTED_EDGE ( 'NONE', *, *, #12910, .F. ) ;
#8201=CARTESIAN_POINT ( 'NONE',  ( 3.231158466157551423, 19.73726462726227737, -35.00000000000000000 ) ) ;
#8210=ORIENTED_EDGE ( 'NONE', *, *, #12297, .F. ) ;
#8235=CIRCLE ( 'NONE', #12449, 20.00000000000001066 ) ;
#8236=CARTESIAN_POINT ( 'NONE',  ( -129.1404785418517918, -15.35070196317932911, -5.500000000000000000 ) ) ;
#8273=ADVANCED_FACE ( 'NONE', ( #7465 ), #17536, .T. ) ;
#8277=FACE_OUTER_BOUND ( 'NONE', #12038, .T. ) ;
#8308=ORIENTED_EDGE ( 'NONE', *, *, #6851, .T. ) ;
#8314=CARTESIAN_POINT ( 'NONE',  ( -128.8626752476364459, 9.172828411137484039, 4.224609204322598899 ) ) ;
#8324=CARTESIAN_POINT ( 'NONE',  ( -84.16800061185418258, 32.38614985672617763, 35.00001200000001234 ) ) ;
#8328=CARTESIAN_POINT ( 'NONE',  ( -90.00000000000000000, 34.99999999999999289, -30.00000000000000355 ) ) ;
#8332=ORIENTED_EDGE ( 'NONE', *, *, #9224, .F. ) ;
#8351=VECTOR ( 'NONE', #4395, 1000.000000000000000 ) ;
#8358=ORIENTED_EDGE ( 'NONE', *, *, #7026, .T. ) ;
#8372=ORIENTED_EDGE ( 'NONE', *, *, #14376, .F. ) ;
#8380=CARTESIAN_POINT ( 'NONE',  ( -129.1404785418517918, -2.850701963179328668, 5.500000000000000000 ) ) ;
#8396=CARTESIAN_POINT ( 'NONE',  ( -105.1664215174088355, -37.48287248576487940, 2.500000000000000000 ) ) ;
#8410=DIRECTION ( 'NONE',  ( -1.000000000000000000, 0.000000000000000000, 0.000000000000000000 ) ) ;
#8423=EDGE_CURVE ( 'NONE', #6209, #3396, #16649, .T. ) ;
#8424=ORIENTED_EDGE ( 'NONE', *, *, #6908, .F. ) ;
#8429=EDGE_LOOP ( 'NONE', ( #14092, #4746, #3986, #9955 ) ) ;
#8438=CARTESIAN_POINT ( 'NONE',  ( -309.1404785418517918, -2.850701963179328668, 9.951701414186818625E-16 ) ) ;
#8457=LINE ( 'NONE', #1274, #17556 ) ;
#8488=VECTOR ( 'NONE', #14524, 1000.000000000000000 ) ;
#8491=FACE_OUTER_BOUND ( 'NONE', #4080, .T. ) ;
#8498=VERTEX_POINT ( 'NONE', #8932 ) ;
#8505=CARTESIAN_POINT ( 'NONE',  ( -127.6870874808773380, 9.532027616443281559, 2.921574671186279559 ) ) ;
#8511=CONICAL_SURFACE ( 'NONE', #14258, 12.74754878398196567, 0.01745329251994333364 ) ;
#8566=ADVANCED_FACE ( 'NONE', ( #9821 ), #8511, .T. ) ;
#8584=EDGE_CURVE ( 'NONE', #9621, #17370, #5566, .T. ) ;
#8592=CARTESIAN_POINT ( 'NONE',  ( -85.86167379012967160, 34.32252072304513746, -35.00000000000000000 ) ) ;
#8601=CARTESIAN_POINT ( 'NONE',  ( -129.0032285637105076, 9.043624184701180013, 4.582591203971080773 ) ) ;
#8624=DIRECTION ( 'NONE',  ( 1.000000000000000000, 0.000000000000000000, 0.000000000000000000 ) ) ;
#8625=DIRECTION ( 'NONE',  ( -0.000000000000000000, -0.000000000000000000, -1.000000000000000000 ) ) ;
#8639=DIRECTION ( 'NONE',  ( 1.000000000000000000, 0.000000000000000000, 0.000000000000000000 ) ) ;
#8648=DIRECTION ( 'NONE',  ( 0.000000000000000000, 0.000000000000000000, -1.000000000000000000 ) ) ;
#8679=CARTESIAN_POINT ( 'NONE',  ( -94.14047854185179176, 6.938893903907228378E-15, 35.00000000000000000 ) ) ;
#8686=DIRECTION ( 'NONE',  ( -0.9998476951563911586, 2.137303368083795934E-18, -0.01745240643728354635 ) ) ;
#8689=DIRECTION ( 'NONE',  ( -0.000000000000000000, -0.000000000000000000, 1.000000000000000000 ) ) ;
#8714=FACE_OUTER_BOUND ( 'NONE', #1761, .T. ) ;
#8723=DIRECTION ( 'NONE',  ( -0.000000000000000000, -0.000000000000000000, 1.000000000000000000 ) ) ;
#8756=CARTESIAN_POINT ( 'NONE',  ( -89.99999999999998579, -35.00000000000001421, 35.00000000000000000 ) ) ;
#8767=CARTESIAN_POINT ( 'NONE',  ( -129.1404785418517918, -15.35070196317932911, 2.500000000000000000 ) ) ;
#8768=ORIENTED_EDGE ( 'NONE', *, *, #10953, .T. ) ;
#8777=CARTESIAN_POINT ( 'NONE',  ( -89.99999999999998579, -35.00000000000001421, -2.500000000000000000 ) ) ;
#8781=CARTESIAN_POINT ( 'NONE',  ( -129.1404785418517918, -2.850701963179328668, 9.951701414186818625E-16 ) ) ;
#8790=CIRCLE ( 'NONE', #4551, 150.0000000000000000 ) ;
#8793=ORIENTED_EDGE ( 'NONE', *, *, #5620, .T. ) ;
#8800=AXIS2_PLACEMENT_3D ( 'NONE', #5257, #9231, #15204 ) ;
#8804=CARTESIAN_POINT ( 'NONE',  ( 0.000000000000000000, 0.000000000000000000, 35.00000000000000000 ) ) ;
#8827=DIRECTION ( 'NONE',  ( -0.9868632313631133801, 0.1615579233078772714, 2.699728182682517290E-16 ) ) ;
#8840=ORIENTED_EDGE ( 'NONE', *, *, #4880, .T. ) ;
#8842=AXIS2_PLACEMENT_3D ( 'NONE', #12883, #8723, #8639 ) ;
#8880=ORIENTED_EDGE ( 'NONE', *, *, #9267, .T. ) ;
#8899=CARTESIAN_POINT ( 'NONE',  ( -84.20693962813486166, 32.64562644091790844, -35.00000000000000000 ) ) ;
#8902=CARTESIAN_POINT ( 'NONE',  ( -128.1404785157144204, 9.631497293019405603, 2.500000000000000000 ) ) ;
#8920=ORIENTED_EDGE ( 'NONE', *, *, #9657, .T. ) ;
#8932=CARTESIAN_POINT ( 'NONE',  ( 2.000000000000000000, 2.449293598294706414E-16, 35.00000000000000000 ) ) ;
#8933=ORIENTED_EDGE ( 'NONE', *, *, #11310, .F. ) ;
#8939=CARTESIAN_POINT ( 'NONE',  ( -126.1404785418517918, -15.29729532696464567, -2.500000000000000000 ) ) ;
#8949=AXIS2_PLACEMENT_3D ( 'NONE', #8438, #7041, #12786 ) ;
#8952=EDGE_CURVE ( 'NONE', #2351, #3748, #12102, .T. ) ;
#8955=( NAMED_UNIT ( * ) SI_UNIT ( $, .STERADIAN. ) SOLID_ANGLE_UNIT ( ) );
#8964=DIRECTION ( 'NONE',  ( -0.000000000000000000, -0.000000000000000000, -1.000000000000000000 ) ) ;
#8966=LINE ( 'NONE', #14754, #14565 ) ;
#8992=DIRECTION ( 'NONE',  ( 1.000000000000000000, 0.000000000000000000, 0.000000000000000000 ) ) ;
#8995=ORIENTED_EDGE ( 'NONE', *, *, #14781, .T. ) ;
#8997=DIRECTION ( 'NONE',  ( -1.000000000000000000, 0.000000000000000000, 0.000000000000000000 ) ) ;
#9013=ORIENTED_EDGE ( 'NONE', *, *, #14350, .F. ) ;
#9054=DIRECTION ( 'NONE',  ( 1.000000000000000000, 0.000000000000000000, 0.000000000000000000 ) ) ;
#9074=FACE_OUTER_BOUND ( 'NONE', #8165, .T. ) ;
#9076=PRODUCT ( 'Lower Hopper Receiver Handle Arm', 'Lower Hopper Receiver Handle Arm', '', ( #4199 ) ) ;
#9091=LINE ( 'NONE', #7490, #11381 ) ;
#9094=CYLINDRICAL_SURFACE ( 'NONE', #12748, 2.000000000000001776 ) ;
#9101=UNCERTAINTY_MEASURE_WITH_UNIT (LENGTH_MEASURE( 1.000000000000000082E-05 ), #7650, 'distance_accuracy_value', 'NONE');
#9105=VERTEX_POINT ( 'NONE', #861 ) ;
#9117=VERTEX_POINT ( 'NONE', #12666 ) ;
#9129=ORIENTED_EDGE ( 'NONE', *, *, #16451, .F. ) ;
#9143=DIRECTION ( 'NONE',  ( -1.000000000000000000, 0.000000000000000000, 0.000000000000000000 ) ) ;
#9158=CIRCLE ( 'NONE', #12939, 12.74754878398196567 ) ;
#9167=ORIENTED_EDGE ( 'NONE', *, *, #7441, .F. ) ;
#9178=ORIENTED_EDGE ( 'NONE', *, *, #10062, .T. ) ;
#9199=CARTESIAN_POINT ( 'NONE',  ( -90.00000000000000000, 34.99999999999999289, 30.00000000000002487 ) ) ;
#9220=DIRECTION ( 'NONE',  ( 0.9868632313631133801, -0.1615579233078772714, 0.000000000000000000 ) ) ;
#9224=EDGE_CURVE ( 'NONE', #12364, #3748, #15997, .T. ) ;
#9231=DIRECTION ( 'NONE',  ( -0.000000000000000000, -0.000000000000000000, -1.000000000000000000 ) ) ;
#9232=AXIS2_PLACEMENT_3D ( 'NONE', #8099, #9625, #14063 ) ;
#9236=SURFACE_STYLE_USAGE ( .BOTH. , #1857 ) ;
#9242=ORIENTED_EDGE ( 'NONE', *, *, #8423, .T. ) ;
#9267=EDGE_CURVE ( 'NONE', #12882, #13318, #1247, .T. ) ;
#9280=CARTESIAN_POINT ( 'NONE',  ( -127.5081579206795936, -15.25292806682357494, -2.822349119005437057 ) ) ;
#9288=VECTOR ( 'NONE', #17558, 1000.000000000000000 ) ;
#9309=CARTESIAN_POINT ( 'NONE',  ( -129.1404785418517918, -15.35070196317932911, 2.500000000000000000 ) ) ;
#9310=EDGE_LOOP ( 'NONE', ( #13626, #15940, #2176, #2624 ) ) ;
#9323=FACE_OUTER_BOUND ( 'NONE', #2316, .T. ) ;
#9339=AXIS2_PLACEMENT_3D ( 'NONE', #11975, #2057, #3654 ) ;
#9344=VECTOR ( 'NONE', #13441, 1000.000000000000000 ) ;
#9347=EDGE_LOOP ( 'NONE', ( #9599, #2674, #8372, #9556 ) ) ;
#9350=LINE ( 'NONE', #3272, #10350 ) ;
#9367=EDGE_LOOP ( 'NONE', ( #3993, #13687, #16979, #6561 ) ) ;
#9368=VERTEX_POINT ( 'NONE', #1873 ) ;
#9374=DIRECTION ( 'NONE',  ( 0.000000000000000000, 0.000000000000000000, 1.000000000000000000 ) ) ;
#9377=CARTESIAN_POINT ( 'NONE',  ( -127.6870874808773664, -15.23343154280193978, -2.921574671186279559 ) ) ;
#9387=EDGE_CURVE ( 'NONE', #13932, #9656, #17083, .T. ) ;
#9388=VECTOR ( 'NONE', #10355, 1000.000000000000114 ) ;
#9403=VECTOR ( 'NONE', #116, 1000.000000000000227 ) ;
#9411=ADVANCED_FACE ( 'NONE', ( #9074 ), #12075, .F. ) ;
#9412=PLANE ( 'NONE',  #3322 ) ;
#9464=EDGE_CURVE ( 'NONE', #16710, #17960, #9749, .T. ) ;
#9478=LINE ( 'NONE', #1070, #7460 ) ;
#9480=CARTESIAN_POINT ( 'NONE',  ( 3.231158466157545206, -19.73726462726228092, 35.00000000000000000 ) ) ;
#9484=FACE_OUTER_BOUND ( 'NONE', #9367, .T. ) ;
#9509=EDGE_CURVE ( 'NONE', #11897, #17960, #11884, .T. ) ;
#9512=ORIENTED_EDGE ( 'NONE', *, *, #5345, .F. ) ;
#9556=ORIENTED_EDGE ( 'NONE', *, *, #10006, .T. ) ;
#9568=DIRECTION ( 'NONE',  ( -0.000000000000000000, -0.000000000000000000, -1.000000000000000000 ) ) ;
#9577=ORIENTED_EDGE ( 'NONE', *, *, #15762, .F. ) ;
#9593=EDGE_CURVE ( 'NONE', #44, #13932, #13782, .T. ) ;
#9599=ORIENTED_EDGE ( 'NONE', *, *, #16451, .T. ) ;
#9613=CYLINDRICAL_SURFACE ( 'NONE', #18558, 150.0000000000000000 ) ;
#9620=DIRECTION ( 'NONE',  ( -3.039628882124824168E-17, -0.000000000000000000, 1.000000000000000000 ) ) ;
#9621=VERTEX_POINT ( 'NONE', #7009 ) ;
#9625=DIRECTION ( 'NONE',  ( 3.039628882124824168E-17, 0.000000000000000000, -1.000000000000000000 ) ) ;
#9628=CYLINDRICAL_SURFACE ( 'NONE', #5139, 2.000000000000000000 ) ;
#9633=AXIS2_PLACEMENT_3D ( 'NONE', #14590, #1616, #7396 ) ;
#9656=VERTEX_POINT ( 'NONE', #15690 ) ;
#9657=EDGE_CURVE ( 'NONE', #3651, #5894, #16630, .T. ) ;
#9665=DIRECTION ( 'NONE',  ( 3.039628882124824168E-17, 0.000000000000000000, -1.000000000000000000 ) ) ;
#9675=CARTESIAN_POINT ( 'NONE',  ( -127.6813802953510333, 9.532733159319212390, -2.918139657044711122 ) ) ;
#9680=VECTOR ( 'NONE', #8161, 1000.000000000000000 ) ;
#9683=ORIENTED_EDGE ( 'NONE', *, *, #10062, .F. ) ;
#9732=CARTESIAN_POINT ( 'NONE',  ( 55.85952145814821534, 6.938893903907228378E-15, 35.00000000000000000 ) ) ;
#9747=ORIENTED_EDGE ( 'NONE', *, *, #16548, .F. ) ;
#9749=LINE ( 'NONE', #12477, #15236 ) ;
#9771=DIRECTION ( 'NONE',  ( 0.000000000000000000, 0.000000000000000000, 1.000000000000000000 ) ) ;
#9777=ORIENTED_EDGE ( 'NONE', *, *, #18780, .F. ) ;
#9791=CARTESIAN_POINT ( 'NONE',  ( 3.231158466157551423, 19.73726462726227737, 35.00000000000000000 ) ) ;
#9794=VERTEX_POINT ( 'NONE', #12614 ) ;
#9799=ORIENTED_EDGE ( 'NONE', *, *, #17051, .F. ) ;
#9801=CARTESIAN_POINT ( 'NONE',  ( -128.8620198725178909, -14.87463575837847962, 4.223374618371430245 ) ) ;
#9810=CARTESIAN_POINT ( 'NONE',  ( -306.1404785418517918, -2.850701963179326892, -12.83663829214475882 ) ) ;
#9816=LINE ( 'NONE', #6120, #18519 ) ;
#9821=FACE_OUTER_BOUND ( 'NONE', #18119, .T. ) ;
#9834=CARTESIAN_POINT ( 'NONE',  ( 55.85952145814821534, 6.938893903907228378E-15, 35.00000000000000000 ) ) ;
#9848=DIRECTION ( 'NONE',  ( -1.000000000000000000, 0.000000000000000000, 0.000000000000000000 ) ) ;
#9866=DIRECTION ( 'NONE',  ( -0.000000000000000000, -0.000000000000000000, -1.000000000000000000 ) ) ;
#9875=EDGE_CURVE ( 'NONE', #3975, #17212, #5537, .T. ) ;
#9882=CARTESIAN_POINT ( 'NONE',  ( 55.85952145814821534, 6.938893903907228378E-15, 29.99999999999998579 ) ) ;
#9893=CYLINDRICAL_SURFACE ( 'NONE', #3762, 5.000000000000004441 ) ;
#9896=CARTESIAN_POINT ( 'NONE',  ( -90.00000000000000000, 34.99999999999999289, 35.00000000000000000 ) ) ;
#9903=EDGE_CURVE ( 'NONE', #44, #8498, #13345, .T. ) ;
#9933=B_SPLINE_CURVE_WITH_KNOTS ( 'NONE', 3,
 ( #12499, #18345, #2470, #5311, #768, #11065, #9675, #6837, #18240, #1153, #15535, #5501, #18337, #5212, #6544, #12289, #18129, #16694 ),
 .UNSPECIFIED., .F., .F.,
 ( 4, 2, 2, 2, 2, 2, 2, 2, 4 ),
 ( 0.000000000000000000, 0.0006036110467293980117, 0.001207222093458796023, 0.001810833140188194360, 0.002414444186917592047, 0.003018055233646990167, 0.003621666280376389154, 0.004225277327105789009, 0.004828888373835187563 ),
 .UNSPECIFIED. ) ;
#9936=LINE ( 'NONE', #15908, #12575 ) ;
#9950=FACE_OUTER_BOUND ( 'NONE', #215, .T. ) ;
#9951=ADVANCED_FACE ( 'NONE', ( #17110 ), #660, .T. ) ;
#9955=ORIENTED_EDGE ( 'NONE', *, *, #9956, .T. ) ;
#9956=EDGE_CURVE ( 'NONE', #17580, #16906, #39, .T. ) ;
#9971=EDGE_LOOP ( 'NONE', ( #17016, #4124, #5937, #13112, #16656, #4786, #11026, #7680, #11544 ) ) ;
#9979=VECTOR ( 'NONE', #15574, 1000.000000000000000 ) ;
#10003=CARTESIAN_POINT ( 'NONE',  ( -129.0554062880559627, 8.972188178592761076, 4.766626691765361912 ) ) ;
#10006=EDGE_CURVE ( 'NONE', #2561, #10528, #3389, .T. ) ;
#10016=AXIS2_PLACEMENT_3D ( 'NONE', #18391, #18089, #5364 ) ;
#10021=ORIENTED_EDGE ( 'NONE', *, *, #4969, .T. ) ;
#10022=ORIENTED_EDGE ( 'NONE', *, *, #17340, .T. ) ;
#10031=PLANE ( 'NONE',  #10530 ) ;
#10040=EDGE_LOOP ( 'NONE', ( #10725, #7170, #6144, #14362, #3027 ) ) ;
#10062=EDGE_CURVE ( 'NONE', #9117, #11762, #14872, .T. ) ;
#10093=CARTESIAN_POINT ( 'NONE',  ( -77.72973689007648090, 30.96463005215034059, -35.00000000000000000 ) ) ;
#10101=DIRECTION ( 'NONE',  ( 1.000000000000000000, 0.000000000000000000, 0.000000000000000000 ) ) ;
#10154=DIRECTION ( 'NONE',  ( 1.000000000000000000, 0.000000000000000000, -2.631994239413086031E-16 ) ) ;
#10186=VECTOR ( 'NONE', #17415, 1000.000000000000114 ) ;
#10192=VERTEX_POINT ( 'NONE', #14104 ) ;
#10210=DIRECTION ( 'NONE',  ( -1.000000000000000000, 0.000000000000000000, 0.000000000000000000 ) ) ;
#10212=DIRECTION ( 'NONE',  ( 0.000000000000000000, 0.000000000000000000, 1.000000000000000000 ) ) ;
#10213=EDGE_CURVE ( 'NONE', #5894, #12413, #8235, .T. ) ;
#10217=DIRECTION ( 'NONE',  ( -1.000000000000000000, 0.000000000000000000, 0.000000000000000000 ) ) ;
#10226=CIRCLE ( 'NONE', #2056, 150.0000000000000000 ) ;
#10249=DIRECTION ( 'NONE',  ( 1.000000000000000000, 0.000000000000000000, 0.000000000000000000 ) ) ;
#10310=VECTOR ( 'NONE', #14658, 1000.000000000000000 ) ;
#10323=VECTOR ( 'NONE', #10386, 1000.000000000000227 ) ;
#10346=ADVANCED_FACE ( 'NONE', ( #16190 ), #10480, .F. ) ;
#10347=ORIENTED_EDGE ( 'NONE', *, *, #17752, .T. ) ;
#10350=VECTOR ( 'NONE', #17727, 1000.000000000000000 ) ;
#10355=DIRECTION ( 'NONE',  ( 0.9868632313631133801, 0.1615579233078775490, -2.699728182682516797E-16 ) ) ;
#10359=ORIENTED_EDGE ( 'NONE', *, *, #148, .F. ) ;
#10360=ORIENTED_EDGE ( 'NONE', *, *, #14331, .T. ) ;
#10374=LINE ( 'NONE', #8777, #13894 ) ;
#10386=DIRECTION ( 'NONE',  ( 0.9723968097209870765, 0.2333333333333371951, -2.660152884942554774E-16 ) ) ;
#10389=DIRECTION ( 'NONE',  ( 0.9723968097209878536, -0.2333333333333339199, 0.000000000000000000 ) ) ;
#10396=EDGE_CURVE ( 'NONE', #18395, #14596, #17347, .T. ) ;
#10401=VERTEX_POINT ( 'NONE', #6155 ) ;
#10404=EDGE_LOOP ( 'NONE', ( #13279, #11170, #12439, #9512, #2197, #16996, #11305, #11147, #2216, #1037 ) ) ;
#10444=CARTESIAN_POINT ( 'NONE',  ( 55.85952145814821534, 6.938893903907228378E-15, -2.500000000000000000 ) ) ;
#10445=EDGE_CURVE ( 'NONE', #11399, #11897, #9350, .T. ) ;
#10457=ORIENTED_EDGE ( 'NONE', *, *, #13737, .F. ) ;
#10460=CARTESIAN_POINT ( 'NONE',  ( -81.73462711737164454, 33.01666666666666572, -35.00000000000000000 ) ) ;
#10478=DIRECTION ( 'NONE',  ( 1.000000000000000000, 0.000000000000000000, 0.000000000000000000 ) ) ;
#10479=AXIS2_PLACEMENT_3D ( 'NONE', #3355, #9620, #15115 ) ;
#10480=PLANE ( 'NONE',  #16127 ) ;
#10481=DIRECTION ( 'NONE',  ( -0.000000000000000000, -0.000000000000000000, 1.000000000000000000 ) ) ;
#10483=FACE_OUTER_BOUND ( 'NONE', #122, .T. ) ;
#10500=VERTEX_POINT ( 'NONE', #1961 ) ;
#10510=CARTESIAN_POINT ( 'NONE',  ( -129.1404785418517918, -14.43865647753341896, -5.316095106350545940 ) ) ;
#10513=DIRECTION ( 'NONE',  ( -0.9868632313631133801, -0.1615579233078773269, 0.000000000000000000 ) ) ;
#10520=CIRCLE ( 'NONE', #9633, 2.000000000000000000 ) ;
#10524=ORIENTED_EDGE ( 'NONE', *, *, #11852, .F. ) ;
#10528=VERTEX_POINT ( 'NONE', #16778 ) ;
#10530=AXIS2_PLACEMENT_3D ( 'NONE', #7391, #16000, #4144 ) ;
#10573=ORIENTED_EDGE ( 'NONE', *, *, #16548, .T. ) ;
#10622=CARTESIAN_POINT ( 'NONE',  ( -129.1404785418517918, -14.35070196317933267, -5.500000000000000000 ) ) ;
#10656=CARTESIAN_POINT ( 'NONE',  ( -90.00000000000000000, 34.99999999999999289, -35.00000000000000000 ) ) ;
#10674=DIRECTION ( 'NONE',  ( 0.9868632313631133801, -0.1615579233078772714, 2.999697980758352134E-17 ) ) ;
#10679=DIRECTION ( 'NONE',  ( 0.000000000000000000, 0.000000000000000000, 1.000000000000000000 ) ) ;
#10686=VERTEX_POINT ( 'NONE', #2979 ) ;
#10707=DIRECTION ( 'NONE',  ( 1.000000000000000000, 0.000000000000000000, 0.000000000000000000 ) ) ;
#10717=FACE_OUTER_BOUND ( 'NONE', #11632, .T. ) ;
#10724=ORIENTED_EDGE ( 'NONE', *, *, #14184, .T. ) ;
#10725=ORIENTED_EDGE ( 'NONE', *, *, #2998, .F. ) ;
#10731=AXIS2_PLACEMENT_3D ( 'NONE', #5775, #16177, #10101 ) ;
#10759=ORIENTED_EDGE ( 'NONE', *, *, #6058, .F. ) ;
#10762=ORIENTED_EDGE ( 'NONE', *, *, #14228, .T. ) ;
#10772=CARTESIAN_POINT ( 'NONE',  ( -128.0167453206627783, -15.18310030011310729, -3.150553392547042808 ) ) ;
#10774=CARTESIAN_POINT ( 'NONE',  ( -89.14047854185180597, 6.938893903907228378E-15, 30.00000000000002487 ) ) ;
#10780=CARTESIAN_POINT ( 'NONE',  ( -129.1404785418517918, 52.54032238931508658, -2.500000000000000000 ) ) ;
#10781=DIRECTION ( 'NONE',  ( 0.000000000000000000, 0.000000000000000000, 1.000000000000000000 ) ) ;
#10790=ORIENTED_EDGE ( 'NONE', *, *, #6908, .T. ) ;
#10802=DIRECTION ( 'NONE',  ( 0.9868632313631133801, -0.1615579233078772714, 0.000000000000000000 ) ) ;
#10819=DIRECTION ( 'NONE',  ( -0.000000000000000000, -0.000000000000000000, -1.000000000000000000 ) ) ;
#10829=CARTESIAN_POINT ( 'NONE',  ( -129.1404785418517918, -2.850701963179328668, 9.951701414186818625E-16 ) ) ;
#10832=ORIENTED_EDGE ( 'NONE', *, *, #10953, .F. ) ;
#10842=AXIS2_PLACEMENT_3D ( 'NONE', #17482, #4473, #13182 ) ;
#10851=CARTESIAN_POINT ( 'NONE',  ( -309.1404785418517918, -2.850701963179328668, 9.951701414186818625E-16 ) ) ;
#10868=CIRCLE ( 'NONE', #5130, 2.000000000000001776 ) ;
#10876=B_SPLINE_CURVE_WITH_KNOTS ( 'NONE', 3,
 ( #2248, #8324, #8131, #11143, #3839, #2449, #17064, #15603, #5386, #11327, #8027, #15429, #11246, #1137, #14193, #5580, #13792, #4034 ),
 .UNSPECIFIED., .F., .F.,
 ( 4, 2, 2, 2, 2, 2, 2, 2, 4 ),
 ( 0.1542941748202715790, 0.2407081638136732704, 0.3271221528070749063, 0.4135361418004766532, 0.4999501307938782890, 0.5863641197872799804, 0.6727781087806816718, 0.7591920977740833631, 0.8456060867674841663 ),
 .UNSPECIFIED. ) ;
#10877=CARTESIAN_POINT ( 'NONE',  ( -126.5488609203928831, -15.30456603905313173, -2.499999999999998668 ) ) ;
#10881=ADVANCED_FACE ( 'NONE', ( #13398 ), #6418, .F. ) ;
#10887=AXIS2_PLACEMENT_3D ( 'NONE', #4642, #4729, #8997 ) ;
#10918=ORIENTED_EDGE ( 'NONE', *, *, #12391, .T. ) ;
#10953=EDGE_CURVE ( 'NONE', #10686, #1614, #15421, .T. ) ;
#10960=ORIENTED_EDGE ( 'NONE', *, *, #13853, .T. ) ;
#10962=ORIENTED_EDGE ( 'NONE', *, *, #13737, .T. ) ;
#10971=CARTESIAN_POINT ( 'NONE',  ( -129.0032285637105360, -14.74502811105983469, -4.582591203971078997 ) ) ;
#11026=ORIENTED_EDGE ( 'NONE', *, *, #2998, .T. ) ;
#11050=AXIS2_PLACEMENT_3D ( 'NONE', #6111, #7628, #9220 ) ;
#11062=DIRECTION ( 'NONE',  ( 1.000000000000000000, 0.000000000000000000, 0.000000000000000000 ) ) ;
#11065=CARTESIAN_POINT ( 'NONE',  ( -127.5060788346647485, 9.551739887561357278, -2.821239268406352085 ) ) ;
#11078=CARTESIAN_POINT ( 'NONE',  ( -90.00000000000000000, 34.99999999999999289, 100.5765140304660861 ) ) ;
#11104=CARTESIAN_POINT ( 'NONE',  ( -126.5450966053943631, -15.30041110265608673, 2.520603730400377884 ) ) ;
#11106=CIRCLE ( 'NONE', #3231, 15.83618137761393463 ) ;
#11110=CARTESIAN_POINT ( 'NONE',  ( -127.1404785156000941, -15.31509901360656478, -2.500000000000000000 ) ) ;
#11123=ORIENTED_EDGE ( 'NONE', *, *, #14249, .T. ) ;
#11143=CARTESIAN_POINT ( 'NONE',  ( -83.85307456958885552, 31.66350799028677798, 35.00001200000000523 ) ) ;
#11147=ORIENTED_EDGE ( 'NONE', *, *, #6843, .T. ) ;
#11170=ORIENTED_EDGE ( 'NONE', *, *, #14835, .T. ) ;
#11173=EDGE_LOOP ( 'NONE', ( #6140, #11200, #16051, #5335 ) ) ;
#11190=AXIS2_PLACEMENT_3D ( 'NONE', #12658, #11334, #17154 ) ;
#11200=ORIENTED_EDGE ( 'NONE', *, *, #9875, .F. ) ;
#11212=DIRECTION ( 'NONE',  ( -1.000000000000000000, 0.000000000000000000, 0.000000000000000000 ) ) ;
#11217=ORIENTED_EDGE ( 'NONE', *, *, #7277, .T. ) ;
#11222=VECTOR ( 'NONE', #4140, 1000.000000000000000 ) ;
#11228=AXIS2_PLACEMENT_3D ( 'NONE', #11473, #1371, #10249 ) ;
#11234=CARTESIAN_POINT ( 'NONE',  ( -129.1404785418517918, 8.649298036820676217, 5.500000000000000000 ) ) ;
#11246=CARTESIAN_POINT ( 'NONE',  ( -80.84224302102266790, 30.66666482925224102, 35.00001199999999812 ) ) ;
#11264=EDGE_CURVE ( 'NONE', #1614, #482, #12637, .T. ) ;
#11265=EDGE_CURVE ( 'NONE', #16485, #10686, #2371, .T. ) ;
#11276=B_SPLINE_CURVE_WITH_KNOTS ( 'NONE', 3,
 ( #804, #12331, #11104, #13962, #2301, #5154, #12618, #13756, #5254, #3891, #5349, #16929, #9801, #6586, #15568, #18573, #18180, #6692 ),
 .UNSPECIFIED., .F., .F.,
 ( 4, 2, 2, 2, 2, 2, 2, 2, 4 ),
 ( 0.000000000000000000, 0.0006036110467293982285, 0.001207222093458796457, 0.001810833140188194794, 0.002414444186917592914, 0.003018055233646991034, 0.003621666280376389588, 0.004225277327105787274, 0.004828888373835185828 ),
 .UNSPECIFIED. ) ;
#11302=ORIENTED_EDGE ( 'NONE', *, *, #2870, .F. ) ;
#11305=ORIENTED_EDGE ( 'NONE', *, *, #17550, .F. ) ;
#11310=EDGE_CURVE ( 'NONE', #3748, #11897, #8129, .T. ) ;
#11313=DIRECTION ( 'NONE',  ( 0.000000000000000000, 0.000000000000000000, -1.000000000000000000 ) ) ;
#11315=CARTESIAN_POINT ( 'NONE',  ( -89.99999999999998579, -35.00000000000001421, 2.500000000000000000 ) ) ;
#11316=CARTESIAN_POINT ( 'NONE',  ( -126.9542992265478887, 9.594132765015094932, 2.584671478510879528 ) ) ;
#11327=CARTESIAN_POINT ( 'NONE',  ( -81.87959193097326249, 30.50711626588064007, 35.00001199999999102 ) ) ;
#11334=DIRECTION ( 'NONE',  ( -0.000000000000000000, -0.000000000000000000, -1.000000000000000000 ) ) ;
#11341=LINE ( 'NONE', #17159, #11222 ) ;
#11371=CARTESIAN_POINT ( 'NONE',  ( 55.85952145814821534, 6.938893903907228378E-15, -35.00000000000000000 ) ) ;
#11381=VECTOR ( 'NONE', #13159, 1000.000000000000114 ) ;
#11387=STYLED_ITEM ( 'NONE', ( #3163 ), #14964 ) ;
#11399=VERTEX_POINT ( 'NONE', #10774 ) ;
#11415=DIRECTION ( 'NONE',  ( -2.735665993912342121E-16, -0.000000000000000000, -1.000000000000000000 ) ) ;
#11439=DIRECTION ( 'NONE',  ( -0.000000000000000000, -0.000000000000000000, -1.000000000000000000 ) ) ;
#11441=ADVANCED_FACE ( 'NONE', ( #1341 ), #12672, .F. ) ;
#11447=ORIENTED_EDGE ( 'NONE', *, *, #669, .F. ) ;
#11467=CARTESIAN_POINT ( 'NONE',  ( 55.85952145814821534, 6.938893903907228378E-15, -35.00000000000000000 ) ) ;
#11471=AXIS2_PLACEMENT_3D ( 'NONE', #2146, #6712, #14282 ) ;
#11473=CARTESIAN_POINT ( 'NONE',  ( 0.000000000000000000, 0.000000000000000000, 35.00000000000000000 ) ) ;
#11483=VECTOR ( 'NONE', #15674, 1000.000000000000114 ) ;
#11495=VECTOR ( 'NONE', #2077, 1000.000000000000000 ) ;
#11504=CARTESIAN_POINT ( 'NONE',  ( -128.7754985213482257, 9.229958444745710366, 4.052748550462855093 ) ) ;
#11537=ORIENTED_EDGE ( 'NONE', *, *, #1877, .F. ) ;
#11544=ORIENTED_EDGE ( 'NONE', *, *, #14376, .T. ) ;
#11547=ORIENTED_EDGE ( 'NONE', *, *, #11264, .F. ) ;
#11592=LINE ( 'NONE', #7364, #10186 ) ;
#11595=ORIENTED_EDGE ( 'NONE', *, *, #12887, .F. ) ;
#11604=CARTESIAN_POINT ( 'NONE',  ( 55.85952145814821534, 6.938893903907228378E-15, 29.99999999999998579 ) ) ;
#11615=EDGE_CURVE ( 'NONE', #12140, #9117, #17547, .T. ) ;
#11618=DIRECTION ( 'NONE',  ( -0.000000000000000000, -0.000000000000000000, -1.000000000000000000 ) ) ;
#11624=CARTESIAN_POINT ( 'NONE',  ( 0.000000000000000000, 0.000000000000000000, 35.00000000000000000 ) ) ;
#11632=EDGE_LOOP ( 'NONE', ( #8840, #17987, #15438, #9577 ) ) ;
#11643=ADVANCED_FACE ( 'NONE', ( #5876 ), #16107, .F. ) ;
#11656=VECTOR ( 'NONE', #5507, 1000.000000000000000 ) ;
#11665=ORIENTED_EDGE ( 'NONE', *, *, #8423, .F. ) ;
#11667=CIRCLE ( 'NONE', #15926, 12.74754878398196567 ) ;
#11668=CARTESIAN_POINT ( 'NONE',  ( -89.99999999999998579, -35.00000000000001421, -35.00000000000000000 ) ) ;
#11686=DIRECTION ( 'NONE',  ( -1.000000000000000000, 0.000000000000000000, 0.000000000000000000 ) ) ;
#11697=ORIENTED_EDGE ( 'NONE', *, *, #16058, .F. ) ;
#11707=ORIENTED_EDGE ( 'NONE', *, *, #13670, .T. ) ;
#11711=ORIENTED_EDGE ( 'NONE', *, *, #8952, .T. ) ;
#11712=ADVANCED_FACE ( 'NONE', ( #11802 ), #17650, .T. ) ;
#11716=CARTESIAN_POINT ( 'NONE',  ( -138.4775067298212718, -42.93618108924343346, -2.500000000000000000 ) ) ;
#11738=ORIENTED_EDGE ( 'NONE', *, *, #12148, .T. ) ;
#11740=CARTESIAN_POINT ( 'NONE',  ( -129.1404785418517918, 52.54032238931508658, 2.500000000000000000 ) ) ;
#11741=ADVANCED_FACE ( 'NONE', ( #10483 ), #16278, .F. ) ;
#11762=VERTEX_POINT ( 'NONE', #4798 ) ;
#11787=ORIENTED_EDGE ( 'NONE', *, *, #6843, .F. ) ;
#11789=AXIS2_PLACEMENT_3D ( 'NONE', #1364, #2671, #8648 ) ;
#11800=SURFACE_SIDE_STYLE ('',( #12079 ) ) ;
#11802=FACE_OUTER_BOUND ( 'NONE', #12093, .T. ) ;
#11804=AXIS2_PLACEMENT_3D ( 'NONE', #2895, #18784, #13220 ) ;
#11829=B_SPLINE_CURVE_WITH_KNOTS ( 'NONE', 3,
 ( #18383, #4097, #11110, #14059 ),
 .UNSPECIFIED., .F., .F.,
 ( 4, 4 ),
 ( 0.000000000000000000, 0.003000475340473869428 ),
 .UNSPECIFIED. ) ;
#11852=EDGE_CURVE ( 'NONE', #3442, #10192, #14947, .T. ) ;
#11875=FILL_AREA_STYLE ('',( #14839 ) ) ;
#11884=CIRCLE ( 'NONE', #7690, 145.0000000000000284 ) ;
#11897=VERTEX_POINT ( 'NONE', #3833 ) ;
#11902=ORIENTED_EDGE ( 'NONE', *, *, #10213, .F. ) ;
#11912=ORIENTED_EDGE ( 'NONE', *, *, #7868, .T. ) ;
#11923=AXIS2_PLACEMENT_3D ( 'NONE', #14929, #12346, #7827 ) ;
#11928=CARTESIAN_POINT ( 'NONE',  ( -90.00000000000000000, 34.99999999999999289, -35.00000000000000000 ) ) ;
#11952=ORIENTED_EDGE ( 'NONE', *, *, #17752, .F. ) ;
#11959=ORIENTED_EDGE ( 'NONE', *, *, #14184, .F. ) ;
#11972=CARTESIAN_POINT ( 'NONE',  ( -81.73462711737164454, 33.01666666666666572, -35.00000000000000000 ) ) ;
#11975=CARTESIAN_POINT ( 'NONE',  ( -129.1404785418517918, -2.850701963179328668, 9.951701414186818625E-16 ) ) ;
#11998=CARTESIAN_POINT ( 'NONE',  ( -89.99999999999998579, -35.00000000000001421, -30.00000000000000000 ) ) ;
#12002=CARTESIAN_POINT ( 'NONE',  ( -128.1677737538113604, -15.15243288452917270, -3.279750847804472347 ) ) ;
#12009=ORIENTED_EDGE ( 'NONE', *, *, #7441, .T. ) ;
#12022=STYLED_ITEM ( 'NONE', ( #4617 ), #16831 ) ;
#12027=VERTEX_POINT ( 'NONE', #7453 ) ;
#12034=COLOUR_RGB ( '', 0.09019608, 0.27058824, 0.51372549) ;
#12038=EDGE_LOOP ( 'NONE', ( #10457, #12120, #13851, #4456 ) ) ;
#12050=DIRECTION ( 'NONE',  ( -0.000000000000000000, -0.000000000000000000, -1.000000000000000000 ) ) ;
#12069=ORIENTED_EDGE ( 'NONE', *, *, #18375, .T. ) ;
#12075=PLANE ( 'NONE',  #2225 ) ;
#12079=SURFACE_STYLE_FILL_AREA ( #16386 ) ;
#12085=LINE ( 'NONE', #17935, #8488 ) ;
#12093=EDGE_LOOP ( 'NONE', ( #1747, #3976 ) ) ;
#12102=LINE ( 'NONE', #11998, #7077 ) ;
#12112=ORIENTED_EDGE ( 'NONE', *, *, #12136, .F. ) ;
#12120=ORIENTED_EDGE ( 'NONE', *, *, #10396, .F. ) ;
#12136=EDGE_CURVE ( 'NONE', #17252, #5489, #10374, .T. ) ;
#12140=VERTEX_POINT ( 'NONE', #4410 ) ;
#12148=EDGE_CURVE ( 'NONE', #9105, #3382, #3893, .T. ) ;
#12172=ADVANCED_FACE ( 'NONE', ( #7921, #15017 ), #4955, .T. ) ;
#12173=DIRECTION ( 'NONE',  ( 2.735665993912342121E-16, 0.000000000000000000, 1.000000000000000000 ) ) ;
#12187=LINE ( 'NONE', #13794, #3880 ) ;
#12198=CARTESIAN_POINT ( 'NONE',  ( 0.000000000000000000, 0.000000000000000000, -35.00000000000000000 ) ) ;
#12213=EDGE_LOOP ( 'NONE', ( #11912, #3579, #13630, #11952 ) ) ;
#12234=VERTEX_POINT ( 'NONE', #7546 ) ;
#12268=CARTESIAN_POINT ( 'NONE',  ( -2.000000000000000000, 0.000000000000000000, 35.00000000000000000 ) ) ;
#12280=B_SPLINE_CURVE_WITH_KNOTS ( 'NONE', 3,
 ( #3036, #10510, #16304, #3391, #10971, #765, #17948, #16589, #6270, #12002, #10772, #9377, #9280, #18135, #10877, #3677 ),
 .UNSPECIFIED., .F., .F.,
 ( 4, 2, 2, 2, 2, 2, 2, 4 ),
 ( 0.000000000000000000, 0.0006035471611761549556, 0.001207094322352309911, 0.001810641483528464867, 0.002414188644704619822, 0.003017735805880774995, 0.003621282967056929734, 0.004828377289409239645 ),
 .UNSPECIFIED. ) ;
#12289=CARTESIAN_POINT ( 'NONE',  ( -129.1237108893556353, 8.819507310261730737, -5.132104245558539724 ) ) ;
#12291=CARTESIAN_POINT ( 'NONE',  ( 3.231158466157545206, -19.73726462726228092, 35.00000000000000000 ) ) ;
#12297=EDGE_CURVE ( 'NONE', #15938, #14768, #10868, .T. ) ;
#12299=CARTESIAN_POINT ( 'NONE',  ( -94.14047854185179176, 6.938893903907228378E-15, -35.00000000000000000 ) ) ;
#12303=EDGE_CURVE ( 'NONE', #9105, #5608, #11829, .T. ) ;
#12317=ORIENTED_EDGE ( 'NONE', *, *, #11310, .T. ) ;
#12325=ADVANCED_FACE ( 'NONE', ( #2311 ), #13972, .F. ) ;
#12331=CARTESIAN_POINT ( 'NONE',  ( -126.3445361634316981, -15.30092830501151369, 2.499999999999999556 ) ) ;
#12346=DIRECTION ( 'NONE',  ( 0.000000000000000000, 0.000000000000000000, 1.000000000000000000 ) ) ;
#12364=VERTEX_POINT ( 'NONE', #6699 ) ;
#12373=DIRECTION ( 'NONE',  ( 0.000000000000000000, 0.000000000000000000, 1.000000000000000000 ) ) ;
#12391=EDGE_CURVE ( 'NONE', #9794, #13473, #2412, .T. ) ;
#12404=ORIENTED_EDGE ( 'NONE', *, *, #12148, .F. ) ;
#12411=CARTESIAN_POINT ( 'NONE',  ( -77.40662104346073136, 32.93835651487657401, 35.00000000000000000 ) ) ;
#12413=VERTEX_POINT ( 'NONE', #8201 ) ;
#12439=ORIENTED_EDGE ( 'NONE', *, *, #3416, .T. ) ;
#12449=AXIS2_PLACEMENT_3D ( 'NONE', #8147, #13915, #11062 ) ;
#12477=CARTESIAN_POINT ( 'NONE',  ( -85.13801595139511846, 33.83333333333333570, 100.5765140304660861 ) ) ;
#12487=ORIENTED_EDGE ( 'NONE', *, *, #12303, .T. ) ;
#12498=CARTESIAN_POINT ( 'NONE',  ( -129.1404785418517918, -2.850701963179328668, 9.951701414186818625E-16 ) ) ;
#12499=CARTESIAN_POINT ( 'NONE',  ( -126.1404785418517918, 9.595891400605989219, -2.500000000000000000 ) ) ;
#12506=LINE ( 'NONE', #12411, #9680 ) ;
#12510=LINE ( 'NONE', #11078, #2616 ) ;
#12516=CARTESIAN_POINT ( 'NONE',  ( -2.000000000000000000, 0.000000000000000000, 35.00000000000000000 ) ) ;
#12539=DIRECTION ( 'NONE',  ( 1.000000000000000000, 0.000000000000000000, 0.000000000000000000 ) ) ;
#12561=CARTESIAN_POINT ( 'NONE',  ( -77.40662104346073136, 32.93835651487657401, -30.00000000000000000 ) ) ;
#12570=AXIS2_PLACEMENT_3D ( 'NONE', #12828, #17220, #1385 ) ;
#12575=VECTOR ( 'NONE', #11439, 1000.000000000000000 ) ;
#12582=CARTESIAN_POINT ( 'NONE',  ( -129.1404785418517918, -2.850701963179328668, 9.951701414186818625E-16 ) ) ;
#12600=DIRECTION ( 'NONE',  ( 0.000000000000000000, 0.000000000000000000, 1.000000000000000000 ) ) ;
#12614=CARTESIAN_POINT ( 'NONE',  ( -129.1404785418517918, -14.35070196317933444, 5.500000000000000000 ) ) ;
#12618=CARTESIAN_POINT ( 'NONE',  ( -127.6813802953510333, -15.23413708567786706, 2.918139657044713342 ) ) ;
#12635=ORIENTED_EDGE ( 'NONE', *, *, #11852, .T. ) ;
#12637=CIRCLE ( 'NONE', #14778, 2.000000000000001776 ) ;
#12639=DIRECTION ( 'NONE',  ( 0.000000000000000000, 0.000000000000000000, 1.000000000000000000 ) ) ;
#12658=CARTESIAN_POINT ( 'NONE',  ( 55.85952145814821534, 6.938893903907228378E-15, 100.5765140304660861 ) ) ;
#12664=LINE ( 'NONE', #2741, #17009 ) ;
#12666=CARTESIAN_POINT ( 'NONE',  ( -2.000000000000000000, 0.000000000000000000, -35.00000000000000000 ) ) ;
#12672=PLANE ( 'NONE',  #5415 ) ;
#12677=DIRECTION ( 'NONE',  ( -0.9998476951563911586, 0.000000000000000000, 0.01745240643728354635 ) ) ;
#12703=CYLINDRICAL_SURFACE ( 'NONE', #11789, 3.000000000000000000 ) ;
#12727=EDGE_CURVE ( 'NONE', #10500, #10528, #16439, .T. ) ;
#12744=ORIENTED_EDGE ( 'NONE', *, *, #10445, .F. ) ;
#12748=AXIS2_PLACEMENT_3D ( 'NONE', #5972, #1707, #8992 ) ;
#12774=VERTEX_POINT ( 'NONE', #3601 ) ;
#12778=PLANE ( 'NONE',  #18257 ) ;
#12780=DIRECTION ( 'NONE',  ( -0.000000000000000000, -0.000000000000000000, -1.000000000000000000 ) ) ;
#12782=DIRECTION ( 'NONE',  ( -0.1615579233078775490, 0.9868632313631133801, 0.000000000000000000 ) ) ;
#12786=DIRECTION ( 'NONE',  ( 0.000000000000000000, 0.000000000000000000, 1.000000000000000000 ) ) ;
#12794=ADVANCED_FACE ( 'NONE', ( #2577 ), #9412, .F. ) ;
#12828=CARTESIAN_POINT ( 'NONE',  ( -306.1404785418517918, -2.850701963179328668, 12.83663829214476237 ) ) ;
#12843=EDGE_LOOP ( 'NONE', ( #305, #8308 ) ) ;
#12864=DIRECTION ( 'NONE',  ( -0.2333333333333372228, 0.9723968097209871875, 0.000000000000000000 ) ) ;
#12867=CARTESIAN_POINT ( 'NONE',  ( -105.9742111339482307, -32.54855632894931716, 2.500000000000000000 ) ) ;
#12878=ORIENTED_EDGE ( 'NONE', *, *, #13670, .F. ) ;
#12882=VERTEX_POINT ( 'NONE', #17299 ) ;
#12883=CARTESIAN_POINT ( 'NONE',  ( -81.73462711737164454, 33.01666666666666572, -35.00000000000000000 ) ) ;
#12885=VERTEX_POINT ( 'NONE', #18651 ) ;
#12887=EDGE_CURVE ( 'NONE', #13318, #3651, #8790, .T. ) ;
#12905=EDGE_CURVE ( 'NONE', #17960, #584, #4283, .T. ) ;
#12910=EDGE_CURVE ( 'NONE', #10192, #17580, #14337, .T. ) ;
#12934=LINE ( 'NONE', #14382, #16882 ) ;
#12939=AXIS2_PLACEMENT_3D ( 'NONE', #12582, #5694, #18442 ) ;
#12948=AXIS2_PLACEMENT_3D ( 'NONE', #12867, #17443, #8624 ) ;
#12950=DIRECTION ( 'NONE',  ( -0.000000000000000000, -0.000000000000000000, -1.000000000000000000 ) ) ;
#12976=AXIS2_PLACEMENT_3D ( 'NONE', #10851, #7848, #12373 ) ;
#13036=CARTESIAN_POINT ( 'NONE',  ( -90.00000000000001421, 34.99999999999999289, 30.00000000000002842 ) ) ;
#13044=CARTESIAN_POINT ( 'NONE',  ( 2.000000000000000000, 2.449293598294706414E-16, -30.00000000000000000 ) ) ;
#13056=FACE_BOUND ( 'NONE', #12843, .T. ) ;
#13107=LINE ( 'NONE', #1656, #8351 ) ;
#13112=ORIENTED_EDGE ( 'NONE', *, *, #18780, .T. ) ;
#13119=DIRECTION ( 'NONE',  ( -0.000000000000000000, -0.000000000000000000, -1.000000000000000000 ) ) ;
#13134=VERTEX_POINT ( 'NONE', #3490 ) ;
#13159=DIRECTION ( 'NONE',  ( -0.9868632313631133801, -0.1615579233078775490, -2.999697980758351518E-17 ) ) ;
#13164=CIRCLE ( 'NONE', #4980, 3.000000000000000888 ) ;
#13170=PLANE ( 'NONE',  #16317 ) ;
#13182=DIRECTION ( 'NONE',  ( 1.000000000000000000, 1.387778780781444492E-15, 0.000000000000000000 ) ) ;
#13207=AXIS2_PLACEMENT_3D ( 'NONE', #6817, #17147, #8410 ) ;
#13209=CIRCLE ( 'NONE', #15635, 2.000000000000000000 ) ;
#13217=FACE_OUTER_BOUND ( 'NONE', #9310, .T. ) ;
#13220=DIRECTION ( 'NONE',  ( -1.000000000000000000, 0.000000000000000000, 0.000000000000000000 ) ) ;
#13227=EDGE_CURVE ( 'NONE', #7533, #13134, #7410, .T. ) ;
#13229=CARTESIAN_POINT ( 'NONE',  ( 55.85952145814821534, 6.938893903907228378E-15, 35.00000000000000000 ) ) ;
#13234=DIRECTION ( 'NONE',  ( 1.000000000000000000, 0.000000000000000000, 0.000000000000000000 ) ) ;
#13239=DIRECTION ( 'NONE',  ( -0.000000000000000000, -0.000000000000000000, -1.000000000000000000 ) ) ;
#13243=CARTESIAN_POINT ( 'NONE',  ( -126.1404785418517918, 6.938893903907228378E-15, 2.500000000000000000 ) ) ;
#13253=VERTEX_POINT ( 'NONE', #16597 ) ;
#13262=VECTOR ( 'NONE', #5624, 1000.000000000000227 ) ;
#13279=ORIENTED_EDGE ( 'NONE', *, *, #6533, .T. ) ;
#13300=APPLICATION_CONTEXT ( 'automotive_design' ) ;
#13318=VERTEX_POINT ( 'NONE', #12299 ) ;
#13334=( LENGTH_UNIT ( ) NAMED_UNIT ( * ) SI_UNIT ( .MILLI., .METRE. ) );
#13345=CIRCLE ( 'NONE', #11228, 2.000000000000000000 ) ;
#13396=LINE ( 'NONE', #7539, #17616 ) ;
#13398=FACE_OUTER_BOUND ( 'NONE', #17966, .T. ) ;
#13400=CARTESIAN_POINT ( 'NONE',  ( -129.1404785418517918, -2.850701963179328668, 9.951701414186818625E-16 ) ) ;
#13401=SURFACE_STYLE_FILL_AREA ( #11875 ) ;
#13419=ORIENTED_EDGE ( 'NONE', *, *, #8952, .F. ) ;
#13428=DIRECTION ( 'NONE',  ( 1.000000000000000000, 0.000000000000000000, 0.000000000000000000 ) ) ;
#13441=DIRECTION ( 'NONE',  ( -0.000000000000000000, -0.000000000000000000, -1.000000000000000000 ) ) ;
#13471=CARTESIAN_POINT ( 'NONE',  ( -85.13801595139511846, 33.83333333333333570, 30.00000000000005329 ) ) ;
#13473=VERTEX_POINT ( 'NONE', #245 ) ;
#13478=ADVANCED_FACE ( 'NONE', ( #18781 ), #6032, .T. ) ;
#13479=DIRECTION ( 'NONE',  ( 1.000000000000000000, 0.000000000000000000, 0.000000000000000000 ) ) ;
#13482=DIRECTION ( 'NONE',  ( 0.000000000000000000, 0.000000000000000000, 1.000000000000000000 ) ) ;
#13507=B_SPLINE_CURVE_WITH_KNOTS ( 'NONE', 3,
 ( #1487, #7275, #15971, #8767 ),
 .UNSPECIFIED., .F., .F.,
 ( 4, 4 ),
 ( 0.000000000000000000, 0.003000475340473870295 ),
 .UNSPECIFIED. ) ;
#13521=CARTESIAN_POINT ( 'NONE',  ( -129.1404785418517918, -2.850701963179328668, 9.951701414186818625E-16 ) ) ;
#13536=CIRCLE ( 'NONE', #17815, 150.0000000000000000 ) ;
#13537=EDGE_CURVE ( 'NONE', #12885, #294, #2263, .T. ) ;
#13554=ADVANCED_FACE ( 'NONE', ( #1860 ), #17805, .F. ) ;
#13584=CIRCLE ( 'NONE', #286, 145.0000000000000284 ) ;
#13606=DIRECTION ( 'NONE',  ( 0.9868632313631133801, -0.1615579233078772714, 0.000000000000000000 ) ) ;
#13610=DIRECTION ( 'NONE',  ( -0.1615579233078775490, 0.9868632313631133801, 0.000000000000000000 ) ) ;
#13611=CARTESIAN_POINT ( 'NONE',  ( 0.000000000000000000, 0.000000000000000000, 0.000000000000000000 ) ) ;
#13626=ORIENTED_EDGE ( 'NONE', *, *, #14968, .F. ) ;
#13630=ORIENTED_EDGE ( 'NONE', *, *, #10213, .T. ) ;
#13635=DIRECTION ( 'NONE',  ( -0.000000000000000000, -0.000000000000000000, -1.000000000000000000 ) ) ;
#13638=DIRECTION ( 'NONE',  ( -0.1615579233078773547, 0.9868632313631134911, 0.000000000000000000 ) ) ;
#13642=CYLINDRICAL_SURFACE ( 'NONE', #3001, 3.000000000000000000 ) ;
#13649=ADVANCED_FACE ( 'NONE', ( #8491, #2514 ), #3809, .F. ) ;
#13670=EDGE_CURVE ( 'NONE', #8498, #44, #13750, .T. ) ;
#13687=ORIENTED_EDGE ( 'NONE', *, *, #5076, .F. ) ;
#13698=ADVANCED_FACE ( 'NONE', ( #3724 ), #9893, .T. ) ;
#13714=DIRECTION ( 'NONE',  ( -0.000000000000000000, -0.000000000000000000, -1.000000000000000000 ) ) ;
#13725=DIRECTION ( 'NONE',  ( 0.000000000000000000, 1.000000000000000000, -0.000000000000000000 ) ) ;
#13737=EDGE_CURVE ( 'NONE', #14596, #13134, #13164, .T. ) ;
#13750=CIRCLE ( 'NONE', #5612, 2.000000000000000000 ) ;
#13756=CARTESIAN_POINT ( 'NONE',  ( -128.0119535342734878, -15.18399252164955548, 3.146712427857099481 ) ) ;
#13773=EDGE_LOOP ( 'NONE', ( #5638, #10790, #10021, #8920 ) ) ;
#13775=AXIS2_PLACEMENT_3D ( 'NONE', #16175, #14836, #14592 ) ;
#13776=VERTEX_POINT ( 'NONE', #8756 ) ;
#13782=LINE ( 'NONE', #12268, #14938 ) ;
#13792=CARTESIAN_POINT ( 'NONE',  ( -79.62936786100797804, 31.64307958360170048, 35.00001199999999812 ) ) ;
#13794=CARTESIAN_POINT ( 'NONE',  ( -126.1404785418517918, 9.649298036820672664, -2.500000000000000000 ) ) ;
#13810=AXIS2_PLACEMENT_3D ( 'NONE', #13229, #8964, #6047 ) ;
#13850=ORIENTED_EDGE ( 'NONE', *, *, #669, .T. ) ;
#13851=ORIENTED_EDGE ( 'NONE', *, *, #6196, .T. ) ;
#13853=EDGE_CURVE ( 'NONE', #482, #15938, #13107, .T. ) ;
#13858=CIRCLE ( 'NONE', #1485, 29.12282187559191016 ) ;
#13861=AXIS2_PLACEMENT_3D ( 'NONE', #16701, #17844, #866 ) ;
#13866=CARTESIAN_POINT ( 'NONE',  ( -129.1404785418517918, -2.850701963179328668, 9.951701414186818625E-16 ) ) ;
#13869=DIRECTION ( 'NONE',  ( -0.000000000000000000, -0.000000000000000000, -1.000000000000000000 ) ) ;
#13894=VECTOR ( 'NONE', #2890, 1000.000000000000114 ) ;
#13915=DIRECTION ( 'NONE',  ( 0.000000000000000000, 0.000000000000000000, 1.000000000000000000 ) ) ;
#13930=ORIENTED_EDGE ( 'NONE', *, *, #17640, .T. ) ;
#13932=VERTEX_POINT ( 'NONE', #16442 ) ;
#13960=ORIENTED_EDGE ( 'NONE', *, *, #17656, .F. ) ;
#13962=CARTESIAN_POINT ( 'NONE',  ( -126.9394941819792280, -15.29082033824380638, 2.601363783521511763 ) ) ;
#13963=AXIS2_PLACEMENT_3D ( 'NONE', #16883, #9665, #6540 ) ;
#13972=PLANE ( 'NONE',  #8171 ) ;
#13985=ADVANCED_FACE ( 'NONE', ( #10717 ), #16517, .F. ) ;
#13989=CARTESIAN_POINT ( 'NONE',  ( -81.73462711737164454, 33.01666666666666572, 30.00000000000002842 ) ) ;
#13991=CARTESIAN_POINT ( 'NONE',  ( 3.231158466157551423, 19.73726462726227737, -30.00000000000000000 ) ) ;
#14036=DIRECTION ( 'NONE',  ( -1.000000000000000000, 0.000000000000000000, 0.000000000000000000 ) ) ;
#14054=ORIENTED_EDGE ( 'NONE', *, *, #9593, .T. ) ;
#14059=CARTESIAN_POINT ( 'NONE',  ( -126.1404785418517918, -15.29729532696464567, -2.500000000000000000 ) ) ;
#14062=DIRECTION ( 'NONE',  ( -0.000000000000000000, -0.000000000000000000, -1.000000000000000000 ) ) ;
#14063=DIRECTION ( 'NONE',  ( -1.000000000000000000, 0.000000000000000000, -3.039628882124824168E-17 ) ) ;
#14064=ORIENTED_EDGE ( 'NONE', *, *, #7277, .F. ) ;
#14092=ORIENTED_EDGE ( 'NONE', *, *, #5274, .T. ) ;
#14102=DIRECTION ( 'NONE',  ( -0.9723968097209870765, -0.2333333333333371951, 0.000000000000000000 ) ) ;
#14104=CARTESIAN_POINT ( 'NONE',  ( -90.00000000000000000, 34.99999999999999289, 30.00000000000002842 ) ) ;
#14110=CARTESIAN_POINT ( 'NONE',  ( 55.85952145814821534, 6.938893903907228378E-15, -35.00000000000000000 ) ) ;
#14129=ADVANCED_FACE ( 'NONE', ( #15539 ), #5221, .T. ) ;
#14147=DIRECTION ( 'NONE',  ( -1.000000000000000000, 0.000000000000000000, 0.000000000000000000 ) ) ;
#14158=CARTESIAN_POINT ( 'NONE',  ( -84.20693962813486166, 32.64562644091790844, -35.00000000000000000 ) ) ;
#14168=CARTESIAN_POINT ( 'NONE',  ( -77.40662104346073136, 32.93835651487657401, 30.00000000000002132 ) ) ;
#14184=EDGE_CURVE ( 'NONE', #14768, #1614, #9478, .T. ) ;
#14191=DIRECTION ( 'NONE',  ( 0.000000000000000000, 0.000000000000000000, 1.000000000000000000 ) ) ;
#14193=CARTESIAN_POINT ( 'NONE',  ( -80.15829819844529425, 31.05859487262427265, 35.00001199999999812 ) ) ;
#14208=FACE_OUTER_BOUND ( 'NONE', #8429, .T. ) ;
#14213=LINE ( 'NONE', #4050, #11656 ) ;
#14225=CIRCLE ( 'NONE', #6978, 42.89102435249441925 ) ;
#14228=EDGE_CURVE ( 'NONE', #3396, #949, #17458, .T. ) ;
#14236=CONICAL_SURFACE ( 'NONE', #4228, 12.74754878398196567, 0.01745329251994333364 ) ;
#14237=DIRECTION ( 'NONE',  ( -1.000000000000000000, 0.000000000000000000, 0.000000000000000000 ) ) ;
#14249=EDGE_CURVE ( 'NONE', #2390, #13318, #1121, .T. ) ;
#14250=VERTEX_POINT ( 'NONE', #3680 ) ;
#14258=AXIS2_PLACEMENT_3D ( 'NONE', #1726, #1124, #12639 ) ;
#14267=EDGE_CURVE ( 'NONE', #5872, #1792, #14213, .T. ) ;
#14273=DIRECTION ( 'NONE',  ( -1.000000000000000000, 0.000000000000000000, 0.000000000000000000 ) ) ;
#14274=EDGE_CURVE ( 'NONE', #13134, #7533, #5939, .T. ) ;
#14282=DIRECTION ( 'NONE',  ( -1.000000000000000000, 0.000000000000000000, 0.000000000000000000 ) ) ;
#14294=DIRECTION ( 'NONE',  ( 1.000000000000000000, 0.000000000000000000, 0.000000000000000000 ) ) ;
#14314=FACE_OUTER_BOUND ( 'NONE', #5670, .T. ) ;
#14317=CARTESIAN_POINT ( 'NONE',  ( 55.85952145814821534, 6.938893903907228378E-15, 2.500000000000000000 ) ) ;
#14328=ORIENTED_EDGE ( 'NONE', *, *, #9903, .F. ) ;
#14331=EDGE_CURVE ( 'NONE', #11762, #9117, #4417, .T. ) ;
#14337=LINE ( 'NONE', #7339, #1256 ) ;
#14350=EDGE_CURVE ( 'NONE', #610, #11762, #9936, .T. ) ;
#14362=ORIENTED_EDGE ( 'NONE', *, *, #5620, .F. ) ;
#14375=CARTESIAN_POINT ( 'NONE',  ( -126.1404785418517918, 9.595891400605990995, 2.500000000000000000 ) ) ;
#14376=EDGE_CURVE ( 'NONE', #2561, #5872, #6559, .T. ) ;
#14382=CARTESIAN_POINT ( 'NONE',  ( -129.1404785418517918, -2.850701963179326892, -12.74754878398196389 ) ) ;
#14398=CARTESIAN_POINT ( 'NONE',  ( -85.13801595139509004, -33.83333333333328596, 100.5765140304660861 ) ) ;
#14407=DIRECTION ( 'NONE',  ( 0.9868632313631133801, -0.1615579233078772714, 2.999697980758352134E-17 ) ) ;
#14410=ORIENTED_EDGE ( 'NONE', *, *, #5274, .F. ) ;
#14420=ADVANCED_FACE ( 'NONE', ( #17166 ), #4149, .T. ) ;
#14422=AXIS2_PLACEMENT_3D ( 'NONE', #11604, #11415, #4411 ) ;
#14425=CARTESIAN_POINT ( 'NONE',  ( -90.00000000000000000, 34.99999999999999289, 30.00000000000002487 ) ) ;
#14428=ORIENTED_EDGE ( 'NONE', *, *, #9267, .F. ) ;
#14432=AXIS2_PLACEMENT_3D ( 'NONE', #13521, #1623, #16294 ) ;
#14443=CIRCLE ( 'NONE', #6290, 12.74754878398196567 ) ;
#14473=ORIENTED_EDGE ( 'NONE', *, *, #273, .T. ) ;
#14491=CARTESIAN_POINT ( 'NONE',  ( 55.85952145814821534, 6.938893903907228378E-15, 100.5765140304660861 ) ) ;
#14524=DIRECTION ( 'NONE',  ( -0.000000000000000000, -0.000000000000000000, -1.000000000000000000 ) ) ;
#14528=EDGE_LOOP ( 'NONE', ( #876, #15651, #14951, #18332 ) ) ;
#14529=ORIENTED_EDGE ( 'NONE', *, *, #17656, .T. ) ;
#14565=VECTOR ( 'NONE', #10674, 1000.000000000000227 ) ;
#14567=DIRECTION ( 'NONE',  ( 1.000000000000000000, 0.000000000000000000, 0.000000000000000000 ) ) ;
#14590=CARTESIAN_POINT ( 'NONE',  ( 0.000000000000000000, 0.000000000000000000, -30.00000000000000000 ) ) ;
#14592=DIRECTION ( 'NONE',  ( 1.000000000000000000, 0.000000000000000000, 0.000000000000000000 ) ) ;
#14594=ORIENTED_EDGE ( 'NONE', *, *, #12905, .T. ) ;
#14596=VERTEX_POINT ( 'NONE', #746 ) ;
#14607=CARTESIAN_POINT ( 'NONE',  ( -79.50968810220766159, 31.87664632526870889, -35.00000000000000000 ) ) ;
#14616=DIRECTION ( 'NONE',  ( 0.000000000000000000, 0.000000000000000000, 1.000000000000000000 ) ) ;
#14649=DIRECTION ( 'NONE',  ( -0.000000000000000000, -0.000000000000000000, 1.000000000000000000 ) ) ;
#14658=DIRECTION ( 'NONE',  ( -0.000000000000000000, -0.000000000000000000, -1.000000000000000000 ) ) ;
#14670=CARTESIAN_POINT ( 'NONE',  ( -86.18478963674542115, 32.34879426031891114, 35.00000000000000000 ) ) ;
#14691=LINE ( 'NONE', #9199, #8139 ) ;
#14695=AXIS2_PLACEMENT_3D ( 'NONE', #678, #2264, #15347 ) ;
#14700=VERTEX_POINT ( 'NONE', #16970 ) ;
#14754=CARTESIAN_POINT ( 'NONE',  ( -90.00000000000000000, 34.99999999999999289, -30.00000000000000000 ) ) ;
#14759=DIRECTION ( 'NONE',  ( 1.000000000000000000, 0.000000000000000000, 0.000000000000000000 ) ) ;
#14768=VERTEX_POINT ( 'NONE', #5858 ) ;
#14773=ORIENTED_EDGE ( 'NONE', *, *, #10396, .T. ) ;
#14778=AXIS2_PLACEMENT_3D ( 'NONE', #15061, #766, #18136 ) ;
#14781=EDGE_CURVE ( 'NONE', #16710, #10192, #15888, .T. ) ;
#14782=B_SPLINE_CURVE_WITH_KNOTS ( 'NONE', 3,
 ( #11234, #7008, #4219, #10003, #8601, #8314, #11504, #5764, #15879, #2713, #2883, #8505, #5569, #11316, #17054, #14375 ),
 .UNSPECIFIED., .F., .F.,
 ( 4, 2, 2, 2, 2, 2, 2, 4 ),
 ( 0.000000000000000000, 0.0006035471611761543051, 0.001207094322352308610, 0.001810641483528462698, 0.002414188644704618088, 0.003017735805880773694, 0.003621282967056928866, 0.004828377289409239645 ),
 .UNSPECIFIED. ) ;
#14819=ORIENTED_EDGE ( 'NONE', *, *, #7868, .F. ) ;
#14832=DIRECTION ( 'NONE',  ( 0.000000000000000000, 0.000000000000000000, 1.000000000000000000 ) ) ;
#14833=EDGE_CURVE ( 'NONE', #12364, #11399, #3799, .T. ) ;
#14835=EDGE_CURVE ( 'NONE', #1680, #14596, #12934, .T. ) ;
#14836=DIRECTION ( 'NONE',  ( 0.000000000000000000, 0.000000000000000000, 1.000000000000000000 ) ) ;
#14839=FILL_AREA_STYLE_COLOUR ( '', #822 ) ;
#14853=( LENGTH_UNIT ( ) NAMED_UNIT ( * ) SI_UNIT ( .MILLI., .METRE. ) );
#14865=CARTESIAN_POINT ( 'NONE',  ( -127.1404785156000941, 9.613695087247908333, 2.500000000000000000 ) ) ;
#14872=CIRCLE ( 'NONE', #65, 2.000000000000000000 ) ;
#14904=ORIENTED_EDGE ( 'NONE', *, *, #14781, .F. ) ;
#14913=DIRECTION ( 'NONE',  ( 0.000000000000000000, 0.000000000000000000, 1.000000000000000000 ) ) ;
#14922=ORIENTED_EDGE ( 'NONE', *, *, #14833, .F. ) ;
#14929=CARTESIAN_POINT ( 'NONE',  ( 55.85952145814821534, 6.938893903907228378E-15, -2.500000000000000000 ) ) ;
#14938=VECTOR ( 'NONE', #5072, 1000.000000000000000 ) ;
#14947=LINE ( 'NONE', #1965, #18494 ) ;
#14951=ORIENTED_EDGE ( 'NONE', *, *, #13537, .F. ) ;
#14955=LINE ( 'NONE', #18027, #1727 ) ;
#14964=MANIFOLD_SOLID_BREP ( 'Fillet4', #3268 ) ;
#14968=EDGE_CURVE ( 'NONE', #18371, #18389, #7485, .T. ) ;
#14969=PRODUCT_DEFINITION_CONTEXT ( 'detailed design', #13300, 'design' ) ;
#14986=DIRECTION ( 'NONE',  ( -0.000000000000000000, -0.000000000000000000, -1.000000000000000000 ) ) ;
#15011=AXIS2_PLACEMENT_3D ( 'NONE', #2554, #16703, #18249 ) ;
#15017=FACE_BOUND ( 'NONE', #3812, .T. ) ;
#15036=( NAMED_UNIT ( * ) PLANE_ANGLE_UNIT ( ) SI_UNIT ( $, .RADIAN. ) );
#15046=CARTESIAN_POINT ( 'NONE',  ( -89.99999999999998579, -35.00000000000001421, 35.00000000000000000 ) ) ;
#15061=CARTESIAN_POINT ( 'NONE',  ( -77.72973689007648090, 30.96463005215034059, -35.00000000000000000 ) ) ;
#15062=PLANE ( 'NONE',  #16050 ) ;
#15066=AXIS2_PLACEMENT_3D ( 'NONE', #7122, #12782, #2908 ) ;
#15088=CARTESIAN_POINT ( 'NONE',  ( -306.0881213225399051, -2.850701963179328668, 9.951701414186818625E-16 ) ) ;
#15092=FACE_OUTER_BOUND ( 'NONE', #10404, .T. ) ;
#15115=DIRECTION ( 'NONE',  ( -1.000000000000000000, -3.469446951953611033E-15, 0.000000000000000000 ) ) ;
#15127=VERTEX_POINT ( 'NONE', #2871 ) ;
#15128=ORIENTED_EDGE ( 'NONE', *, *, #6644, .F. ) ;
#15143=ORIENTED_EDGE ( 'NONE', *, *, #1852, .T. ) ;
#15165=CARTESIAN_POINT ( 'NONE',  ( -85.86167379012967160, 34.32252072304513746, -30.00000000000000000 ) ) ;
#15172=ORIENTED_EDGE ( 'NONE', *, *, #3201, .F. ) ;
#15189=DIRECTION ( 'NONE',  ( -0.1615579233078772992, -0.9868632313631134911, 0.000000000000000000 ) ) ;
#15191=CARTESIAN_POINT ( 'NONE',  ( -89.99999999999998579, -35.00000000000001421, 100.5765140304660861 ) ) ;
#15201=CARTESIAN_POINT ( 'NONE',  ( -89.99999999999998579, -35.00000000000001421, -35.00000000000000000 ) ) ;
#15204=DIRECTION ( 'NONE',  ( -1.000000000000000000, 0.000000000000000000, 0.000000000000000000 ) ) ;
#15224=ORIENTED_EDGE ( 'NONE', *, *, #16102, .T. ) ;
#15236=VECTOR ( 'NONE', #16863, 1000.000000000000000 ) ;
#15326=DIRECTION ( 'NONE',  ( -0.000000000000000000, -0.000000000000000000, -1.000000000000000000 ) ) ;
#15332=EDGE_CURVE ( 'NONE', #12882, #16906, #8169, .T. ) ;
#15335=AXIS2_PLACEMENT_3D ( 'NONE', #11716, #4540, #13428 ) ;
#15345=DIRECTION ( 'NONE',  ( 0.000000000000000000, 0.000000000000000000, 1.000000000000000000 ) ) ;
#15347=DIRECTION ( 'NONE',  ( 0.000000000000000000, 0.000000000000000000, 1.000000000000000000 ) ) ;
#15355=ORIENTED_EDGE ( 'NONE', *, *, #12910, .T. ) ;
#15398=CARTESIAN_POINT ( 'NONE',  ( 0.000000000000000000, 0.000000000000000000, 35.00000000000000000 ) ) ;
#15404=CYLINDRICAL_SURFACE ( 'NONE', #11471, 20.00000000000001066 ) ;
#15421=CIRCLE ( 'NONE', #4815, 2.500000000000002220 ) ;
#15429=CARTESIAN_POINT ( 'NONE',  ( -81.09522717867928066, 30.58561221855817891, 35.00001199999999812 ) ) ;
#15435=DIRECTION ( 'NONE',  ( -0.000000000000000000, -0.000000000000000000, -1.000000000000000000 ) ) ;
#15437=EDGE_LOOP ( 'NONE', ( #11547, #11959, #8210, #7069 ) ) ;
#15438=ORIENTED_EDGE ( 'NONE', *, *, #4573, .T. ) ;
#15500=DIRECTION ( 'NONE',  ( 0.000000000000000000, 0.000000000000000000, 1.000000000000000000 ) ) ;
#15504=EDGE_CURVE ( 'NONE', #17370, #5489, #1000, .T. ) ;
#15535=CARTESIAN_POINT ( 'NONE',  ( -128.5628356445764382, 9.332895270846938374, -3.719291248522909488 ) ) ;
#15537=DIRECTION ( 'NONE',  ( -0.000000000000000000, -0.000000000000000000, -1.000000000000000000 ) ) ;
#15539=FACE_OUTER_BOUND ( 'NONE', #668, .T. ) ;
#15542=VECTOR ( 'NONE', #17269, 1000.000000000000000 ) ;
#15568=CARTESIAN_POINT ( 'NONE',  ( -129.0548615328497419, -14.67457578939283103, 4.764204982952881196 ) ) ;
#15574=DIRECTION ( 'NONE',  ( -0.000000000000000000, 1.000000000000000000, -0.000000000000000000 ) ) ;
#15578=FACE_OUTER_BOUND ( 'NONE', #10040, .T. ) ;
#15579=DIRECTION ( 'NONE',  ( 0.000000000000000000, -1.445602896647338917E-16, 1.000000000000000000 ) ) ;
#15603=CARTESIAN_POINT ( 'NONE',  ( -82.64970099990441099, 30.67540679198930320, 35.00001199999999812 ) ) ;
#15621=ADVANCED_FACE ( 'NONE', ( #2941 ), #12703, .F. ) ;
#15635=AXIS2_PLACEMENT_3D ( 'NONE', #6074, #4544, #1978 ) ;
#15651=ORIENTED_EDGE ( 'NONE', *, *, #4288, .F. ) ;
#15657=DIRECTION ( 'NONE',  ( -2.735665993912342121E-16, -0.000000000000000000, -1.000000000000000000 ) ) ;
#15673=ORIENTED_EDGE ( 'NONE', *, *, #4550, .T. ) ;
#15674=DIRECTION ( 'NONE',  ( -0.9868632313631133801, 0.1615579233078772436, -0.000000000000000000 ) ) ;
#15690=CARTESIAN_POINT ( 'NONE',  ( 2.000000000000000000, 2.449293598294706414E-16, 30.00000000000000000 ) ) ;
#15696=CARTESIAN_POINT ( 'NONE',  ( -309.1404785418517918, -2.850701963179328668, 9.951701414186818625E-16 ) ) ;
#15705=EDGE_CURVE ( 'NONE', #5872, #12885, #29, .T. ) ;
#15736=ORIENTED_EDGE ( 'NONE', *, *, #9875, .T. ) ;
#15762=EDGE_CURVE ( 'NONE', #584, #2390, #12085, .T. ) ;
#15785=ORIENTED_EDGE ( 'NONE', *, *, #16677, .T. ) ;
#15848=LINE ( 'NONE', #14425, #13262 ) ;
#15879=CARTESIAN_POINT ( 'NONE',  ( -128.4427290061107385, 9.376024958400087428, 3.566331213966848601 ) ) ;
#15888=LINE ( 'NONE', #13036, #4720 ) ;
#15900=CARTESIAN_POINT ( 'NONE',  ( 3.231158466157554976, 19.73726462726227382, 30.00000000000000000 ) ) ;
#15908=CARTESIAN_POINT ( 'NONE',  ( 2.000000000000000000, 2.449293598294706414E-16, 35.00000000000000000 ) ) ;
#15910=CARTESIAN_POINT ( 'NONE',  ( -129.1404785418517918, -2.850701963179328668, 12.74754878398196745 ) ) ;
#15923=AXIS2_PLACEMENT_3D ( 'NONE', #14110, #9771, #18534 ) ;
#15926=AXIS2_PLACEMENT_3D ( 'NONE', #986, #7973, #16810 ) ;
#15938=VERTEX_POINT ( 'NONE', #12561 ) ;
#15940=ORIENTED_EDGE ( 'NONE', *, *, #1975, .F. ) ;
#15971=CARTESIAN_POINT ( 'NONE',  ( -128.1404785157144204, -15.33290121937809403, 2.500000000000000000 ) ) ;
#15974=EDGE_CURVE ( 'NONE', #16318, #294, #10876, .T. ) ;
#15982=ORIENTED_EDGE ( 'NONE', *, *, #15974, .T. ) ;
#15989=EDGE_CURVE ( 'NONE', #9368, #17205, #6918, .T. ) ;
#15992=AXIS2_PLACEMENT_3D ( 'NONE', #14670, #10679, #1875 ) ;
#15997=LINE ( 'NONE', #14398, #15542 ) ;
#16000=DIRECTION ( 'NONE',  ( 2.735665993912342121E-16, 0.000000000000000000, 1.000000000000000000 ) ) ;
#16004=DIRECTION ( 'NONE',  ( 1.000000000000000000, 0.000000000000000000, 0.000000000000000000 ) ) ;
#16013=ORIENTED_EDGE ( 'NONE', *, *, #9593, .F. ) ;
#16034=AXIS2_PLACEMENT_3D ( 'NONE', #11624, #17449, #10217 ) ;
#16050=AXIS2_PLACEMENT_3D ( 'NONE', #2083, #2154, #13606 ) ;
#16051=ORIENTED_EDGE ( 'NONE', *, *, #273, .F. ) ;
#16058=EDGE_CURVE ( 'NONE', #14768, #18371, #3330, .T. ) ;
#16101=CARTESIAN_POINT ( 'NONE',  ( 0.000000000000000000, 0.000000000000000000, 30.00000000000000000 ) ) ;
#16102=EDGE_CURVE ( 'NONE', #8498, #9656, #2726, .T. ) ;
#16107=CYLINDRICAL_SURFACE ( 'NONE', #17545, 145.0000000000000284 ) ;
#16127=AXIS2_PLACEMENT_3D ( 'NONE', #7942, #13610, #7844 ) ;
#16175=CARTESIAN_POINT ( 'NONE',  ( 55.85952145814821534, 6.938893903907228378E-15, 35.00000000000000000 ) ) ;
#16177=DIRECTION ( 'NONE',  ( -0.000000000000000000, -0.000000000000000000, 1.000000000000000000 ) ) ;
#16190=FACE_OUTER_BOUND ( 'NONE', #17918, .T. ) ;
#16200=ORIENTED_EDGE ( 'NONE', *, *, #4288, .T. ) ;
#16220=AXIS2_PLACEMENT_3D ( 'NONE', #870, #1255, #6745 ) ;
#16222=ORIENTED_EDGE ( 'NONE', *, *, #9903, .T. ) ;
#16253=DIRECTION ( 'NONE',  ( -0.9868632313631133801, 0.1615579233078772436, -0.000000000000000000 ) ) ;
#16274=DIRECTION ( 'NONE',  ( -0.2333333333333339477, -0.9723968097209879646, 0.000000000000000000 ) ) ;
#16278=PLANE ( 'NONE',  #9339 ) ;
#16294=DIRECTION ( 'NONE',  ( 0.000000000000000000, 0.000000000000000000, 1.000000000000000000 ) ) ;
#16304=CARTESIAN_POINT ( 'NONE',  ( -129.1237011781999797, -14.52069893526757127, -5.132545408516867802 ) ) ;
#16307=CARTESIAN_POINT ( 'NONE',  ( -84.20693962813486166, 32.64562644091790844, -30.00000000000000355 ) ) ;
#16317=AXIS2_PLACEMENT_3D ( 'NONE', #11467, #17301, #198 ) ;
#16318=VERTEX_POINT ( 'NONE', #2421 ) ;
#16381=VECTOR ( 'NONE', #11313, 1000.000000000000000 ) ;
#16386=FILL_AREA_STYLE ('',( #551 ) ) ;
#16439=LINE ( 'NONE', #3420, #9388 ) ;
#16442=CARTESIAN_POINT ( 'NONE',  ( -2.000000000000000000, 0.000000000000000000, 30.00000000000000000 ) ) ;
#16443=DIRECTION ( 'NONE',  ( 0.000000000000000000, 0.000000000000000000, 1.000000000000000000 ) ) ;
#16451=EDGE_CURVE ( 'NONE', #10528, #1792, #5179, .T. ) ;
#16483=ORIENTED_EDGE ( 'NONE', *, *, #9464, .T. ) ;
#16485=VERTEX_POINT ( 'NONE', #8592 ) ;
#16517=PLANE ( 'NONE',  #11050 ) ;
#16546=ORIENTED_EDGE ( 'NONE', *, *, #4969, .F. ) ;
#16548=EDGE_CURVE ( 'NONE', #3382, #17212, #13858, .T. ) ;
#16589=CARTESIAN_POINT ( 'NONE',  ( -128.5664531142840872, -15.03275830328938945, -3.724467847532855647 ) ) ;
#16592=FACE_OUTER_BOUND ( 'NONE', #6800, .T. ) ;
#16596=DIRECTION ( 'NONE',  ( 1.000000000000000000, 0.000000000000000000, 0.000000000000000000 ) ) ;
#16597=CARTESIAN_POINT ( 'NONE',  ( -126.1404785418517918, -15.29729532696464922, 2.500000000000000000 ) ) ;
#16606=AXIS2_PLACEMENT_3D ( 'NONE', #18246, #9568, #1900 ) ;
#16624=ORIENTED_EDGE ( 'NONE', *, *, #17640, .F. ) ;
#16630=LINE ( 'NONE', #15201, #4871 ) ;
#16649=CIRCLE ( 'NONE', #7562, 2.500000000000002220 ) ;
#16652=DIRECTION ( 'NONE',  ( -1.000000000000000000, 0.000000000000000000, 0.000000000000000000 ) ) ;
#16656=ORIENTED_EDGE ( 'NONE', *, *, #978, .T. ) ;
#16674=PRODUCT_DEFINITION_SHAPE ( 'NONE', 'NONE',  #8012 ) ;
#16677=EDGE_CURVE ( 'NONE', #5722, #17580, #569, .T. ) ;
#16694=CARTESIAN_POINT ( 'NONE',  ( -129.1404785418517918, 8.649298036820674440, -5.500000000000000000 ) ) ;
#16701=CARTESIAN_POINT ( 'NONE',  ( -86.18478963674542115, 32.34879426031891114, -35.00000000000000000 ) ) ;
#16703=DIRECTION ( 'NONE',  ( -0.000000000000000000, -0.000000000000000000, -1.000000000000000000 ) ) ;
#16710=VERTEX_POINT ( 'NONE', #13471 ) ;
#16718=ORIENTED_EDGE ( 'NONE', *, *, #127, .T. ) ;
#16749=DIRECTION ( 'NONE',  ( -3.039628882124824168E-17, -0.000000000000000000, 1.000000000000000000 ) ) ;
#16778=CARTESIAN_POINT ( 'NONE',  ( 3.231158466157545206, -19.73726462726228092, 30.00000000000000000 ) ) ;
#16809=ORIENTED_EDGE ( 'NONE', *, *, #17837, .T. ) ;
#16810=DIRECTION ( 'NONE',  ( 0.000000000000000000, 0.000000000000000000, 1.000000000000000000 ) ) ;
#16831=ADVANCED_BREP_SHAPE_REPRESENTATION ( '', ( #14964, #18772 ), #5087 ) ;
#16839=FACE_OUTER_BOUND ( 'NONE', #2502, .T. ) ;
#16863=DIRECTION ( 'NONE',  ( -0.000000000000000000, -0.000000000000000000, -1.000000000000000000 ) ) ;
#16882=VECTOR ( 'NONE', #8686, 1000.000000000000114 ) ;
#16883=CARTESIAN_POINT ( 'NONE',  ( 0.000000000000000000, 0.000000000000000000, -30.00000000000000000 ) ) ;
#16906=VERTEX_POINT ( 'NONE', #1184 ) ;
#16929=CARTESIAN_POINT ( 'NONE',  ( -128.7747222983995528, -14.93194821374235559, 4.051035741711868532 ) ) ;
#16950=ORIENTED_EDGE ( 'NONE', *, *, #8584, .F. ) ;
#16953=VECTOR ( 'NONE', #7577, 1000.000000000000000 ) ;
#16970=CARTESIAN_POINT ( 'NONE',  ( -126.1404785418517918, 9.595891400605989219, -2.500000000000000000 ) ) ;
#16971=FACE_OUTER_BOUND ( 'NONE', #4608, .T. ) ;
#16979=ORIENTED_EDGE ( 'NONE', *, *, #787, .F. ) ;
#16985=CARTESIAN_POINT ( 'NONE',  ( -129.1404785418517918, 52.54032238931508658, 2.500000000000000000 ) ) ;
#16996=ORIENTED_EDGE ( 'NONE', *, *, #1355, .T. ) ;
#17009=VECTOR ( 'NONE', #2637, 1000.000000000000000 ) ;
#17015=VECTOR ( 'NONE', #1287, 1000.000000000000000 ) ;
#17016=ORIENTED_EDGE ( 'NONE', *, *, #15705, .T. ) ;
#17017=AXIS2_PLACEMENT_3D ( 'NONE', #2123, #716, #6497 ) ;
#17051=EDGE_CURVE ( 'NONE', #12234, #10192, #15848, .T. ) ;
#17054=CARTESIAN_POINT ( 'NONE',  ( -126.5488609203928831, 9.603162112694475283, 2.499999999999999112 ) ) ;
#17062=CYLINDRICAL_SURFACE ( 'NONE', #13207, 2.000000000000000000 ) ;
#17064=CARTESIAN_POINT ( 'NONE',  ( -83.11589401185503334, 30.91643816065307959, 35.00001200000000523 ) ) ;
#17083=CIRCLE ( 'NONE', #1043, 2.000000000000000000 ) ;
#17110=FACE_OUTER_BOUND ( 'NONE', #3074, .T. ) ;
#17114=ORIENTED_EDGE ( 'NONE', *, *, #4948, .T. ) ;
#17131=ORIENTED_EDGE ( 'NONE', *, *, #7403, .F. ) ;
#17142=CIRCLE ( 'NONE', #14695, 12.74754878398196567 ) ;
#17147=DIRECTION ( 'NONE',  ( -0.000000000000000000, -0.000000000000000000, -1.000000000000000000 ) ) ;
#17150=AXIS2_PLACEMENT_3D ( 'NONE', #8804, #10212, #7395 ) ;
#17154=DIRECTION ( 'NONE',  ( -1.000000000000000000, 0.000000000000000000, 0.000000000000000000 ) ) ;
#17159=CARTESIAN_POINT ( 'NONE',  ( -89.99999999999998579, -35.00000000000001421, 100.5765140304660861 ) ) ;
#17166=FACE_OUTER_BOUND ( 'NONE', #8108, .T. ) ;
#17205=VERTEX_POINT ( 'NONE', #10622 ) ;
#17212=VERTEX_POINT ( 'NONE', #18258 ) ;
#17220=DIRECTION ( 'NONE',  ( 0.000000000000000000, -1.000000000000000000, 0.000000000000000000 ) ) ;
#17252=VERTEX_POINT ( 'NONE', #18048 ) ;
#17269=DIRECTION ( 'NONE',  ( -0.000000000000000000, -0.000000000000000000, -1.000000000000000000 ) ) ;
#17276=ADVANCED_FACE ( 'NONE', ( #9484 ), #13642, .F. ) ;
#17299=CARTESIAN_POINT ( 'NONE',  ( -94.14047854185179176, 6.938893903907228378E-15, -2.500000000000000000 ) ) ;
#17301=DIRECTION ( 'NONE',  ( 0.000000000000000000, 0.000000000000000000, 1.000000000000000000 ) ) ;
#17328=DIRECTION ( 'NONE',  ( 1.000000000000000000, 0.000000000000000000, 0.000000000000000000 ) ) ;
#17340=EDGE_CURVE ( 'NONE', #949, #12885, #12506, .T. ) ;
#17347=CIRCLE ( 'NONE', #2492, 15.83618137761393463 ) ;
#17370=VERTEX_POINT ( 'NONE', #2477 ) ;
#17415=DIRECTION ( 'NONE',  ( -0.9868632313631133801, 0.1615579233078772436, -0.000000000000000000 ) ) ;
#17443=DIRECTION ( 'NONE',  ( 0.000000000000000000, 0.000000000000000000, 1.000000000000000000 ) ) ;
#17449=DIRECTION ( 'NONE',  ( -0.000000000000000000, -0.000000000000000000, -1.000000000000000000 ) ) ;
#17458=CIRCLE ( 'NONE', #16220, 2.000000000000001776 ) ;
#17482=CARTESIAN_POINT ( 'NONE',  ( -105.9742111339482307, -32.54855632894931716, -2.500000000000000000 ) ) ;
#17495=CARTESIAN_POINT ( 'NONE',  ( -84.20693962813486166, 32.64562644091790844, 30.00000000000002842 ) ) ;
#17504=ORIENTED_EDGE ( 'NONE', *, *, #14350, .T. ) ;
#17507=FACE_OUTER_BOUND ( 'NONE', #14528, .T. ) ;
#17513=FACE_OUTER_BOUND ( 'NONE', #6706, .T. ) ;
#17520=DIRECTION ( 'NONE',  ( -0.9723968097209878536, 0.2333333333333339199, 2.660152884942556746E-16 ) ) ;
#17536=CYLINDRICAL_SURFACE ( 'NONE', #13810, 150.0000000000000000 ) ;
#17545=AXIS2_PLACEMENT_3D ( 'NONE', #14491, #4527, #10210 ) ;
#17547=LINE ( 'NONE', #5794, #7833 ) ;
#17550=EDGE_CURVE ( 'NONE', #15127, #12774, #1150, .T. ) ;
#17552=CARTESIAN_POINT ( 'NONE',  ( -89.99999999999998579, -35.00000000000001421, 35.00000000000000000 ) ) ;
#17556=VECTOR ( 'NONE', #5616, 1000.000000000000000 ) ;
#17558=DIRECTION ( 'NONE',  ( 0.000000000000000000, -1.000000000000000000, 0.000000000000000000 ) ) ;
#17565=ORIENTED_EDGE ( 'NONE', *, *, #15504, .T. ) ;
#17580=VERTEX_POINT ( 'NONE', #7319 ) ;
#17584=ORIENTED_EDGE ( 'NONE', *, *, #3201, .T. ) ;
#17614=DIRECTION ( 'NONE',  ( 1.000000000000000000, 0.000000000000000000, 0.000000000000000000 ) ) ;
#17616=VECTOR ( 'NONE', #13119, 1000.000000000000000 ) ;
#17633=ORIENTED_EDGE ( 'NONE', *, *, #12391, .F. ) ;
#17640=EDGE_CURVE ( 'NONE', #12774, #13253, #5963, .T. ) ;
#17648=( NAMED_UNIT ( * ) SI_UNIT ( $, .STERADIAN. ) SOLID_ANGLE_UNIT ( ) );
#17650=PLANE ( 'NONE',  #12976 ) ;
#17653=LINE ( 'NONE', #17552, #5355 ) ;
#17656=EDGE_CURVE ( 'NONE', #9105, #3975, #2924, .T. ) ;
#17710=DIRECTION ( 'NONE',  ( 1.000000000000000000, 0.000000000000000000, 0.000000000000000000 ) ) ;
#17711=DIRECTION ( 'NONE',  ( 0.9868632313631133801, -0.1615579233078772714, 0.000000000000000000 ) ) ;
#17727=DIRECTION ( 'NONE',  ( -0.000000000000000000, -0.000000000000000000, -1.000000000000000000 ) ) ;
#17752=EDGE_CURVE ( 'NONE', #1312, #12413, #14955, .T. ) ;
#17756=PLANE ( 'NONE',  #5068 ) ;
#17788=CIRCLE ( 'NONE', #14432, 12.74754878398196567 ) ;
#17805=PLANE ( 'NONE',  #11923 ) ;
#17815=AXIS2_PLACEMENT_3D ( 'NONE', #6181, #769, #2084 ) ;
#17837=EDGE_CURVE ( 'NONE', #12413, #482, #11592, .T. ) ;
#17840=DIRECTION ( 'NONE',  ( 0.9723968097209870765, 0.2333333333333372228, 0.000000000000000000 ) ) ;
#17844=DIRECTION ( 'NONE',  ( -0.000000000000000000, -0.000000000000000000, -1.000000000000000000 ) ) ;
#17847=CARTESIAN_POINT ( 'NONE',  ( -306.0881213225399051, -2.850701963179328668, 15.83618137761393463 ) ) ;
#17876=SHAPE_REPRESENTATION ( 'Lower Hopper Receiver Handle Arm', ( #18772 ), #5087 ) ;
#17888=DIRECTION ( 'NONE',  ( -0.000000000000000000, -0.000000000000000000, -1.000000000000000000 ) ) ;
#17897=ORIENTED_EDGE ( 'NONE', *, *, #17550, .T. ) ;
#17901=DIRECTION ( 'NONE',  ( -1.000000000000000000, 0.000000000000000000, 0.000000000000000000 ) ) ;
#17902=LINE ( 'NONE', #10656, #5118 ) ;
#17918=EDGE_LOOP ( 'NONE', ( #4938, #5801, #1685, #6261 ) ) ;
#17935=CARTESIAN_POINT ( 'NONE',  ( -90.00000000000000000, 34.99999999999999289, 35.00000000000000000 ) ) ;
#17948=CARTESIAN_POINT ( 'NONE',  ( -128.7754985213481689, -14.93136237110436859, -4.052748550462855093 ) ) ;
#17960=VERTEX_POINT ( 'NONE', #4210 ) ;
#17966=EDGE_LOOP ( 'NONE', ( #5910, #10022, #1286, #7045 ) ) ;
#17987=ORIENTED_EDGE ( 'NONE', *, *, #1733, .T. ) ;
#18023=DIRECTION ( 'NONE',  ( 0.000000000000000000, 1.000000000000000000, -0.000000000000000000 ) ) ;
#18027=CARTESIAN_POINT ( 'NONE',  ( 3.231158466157551423, 19.73726462726227737, 35.00000000000000000 ) ) ;
#18037=DIRECTION ( 'NONE',  ( 1.000000000000000000, 0.000000000000000000, 0.000000000000000000 ) ) ;
#18038=UNCERTAINTY_MEASURE_WITH_UNIT (LENGTH_MEASURE( 1.000000000000000082E-05 ), #13334, 'distance_accuracy_value', 'NONE');
#18048=CARTESIAN_POINT ( 'NONE',  ( -105.1664215174088213, -37.48287248576487940, -2.500000000000000000 ) ) ;
#18050=ORIENTED_EDGE ( 'NONE', *, *, #11615, .T. ) ;
#18053=AXIS2_PLACEMENT_3D ( 'NONE', #8006, #2038, #9054 ) ;
#18062=DIRECTION ( 'NONE',  ( -0.000000000000000000, -0.000000000000000000, -1.000000000000000000 ) ) ;
#18078=CYLINDRICAL_SURFACE ( 'NONE', #8800, 29.12282187559192437 ) ;
#18089=DIRECTION ( 'NONE',  ( 2.735665993912342121E-16, 0.000000000000000000, 1.000000000000000000 ) ) ;
#18093=VERTEX_POINT ( 'NONE', #4863 ) ;
#18119=EDGE_LOOP ( 'NONE', ( #6579, #7501, #3023, #3519, #11738, #14064, #12009, #17584, #6809, #14773 ) ) ;
#18129=CARTESIAN_POINT ( 'NONE',  ( -129.1404785418517918, 8.737237296935983721, -5.316127001577083178 ) ) ;
#18135=CARTESIAN_POINT ( 'NONE',  ( -126.9542992265479739, -15.29553669137375671, -2.584671478510880416 ) ) ;
#18136=DIRECTION ( 'NONE',  ( 1.000000000000000000, -3.469446951953611033E-15, 0.000000000000000000 ) ) ;
#18174=CIRCLE ( 'NONE', #10842, 5.000000000000004441 ) ;
#18180=CARTESIAN_POINT ( 'NONE',  ( -129.1404785418518202, -14.43864122329464195, 5.316127001577084066 ) ) ;
#18199=AXIS2_PLACEMENT_3D ( 'NONE', #13400, #4875, #4682 ) ;
#18240=CARTESIAN_POINT ( 'NONE',  ( -128.1659926135409933, 9.451401928990495804, -3.278196957010496959 ) ) ;
#18246=CARTESIAN_POINT ( 'NONE',  ( 55.85952145814821534, 6.938893903907228378E-15, -30.00000000000000000 ) ) ;
#18249=DIRECTION ( 'NONE',  ( -1.000000000000000000, 0.000000000000000000, 0.000000000000000000 ) ) ;
#18257=AXIS2_PLACEMENT_3D ( 'NONE', #86, #12864, #14102 ) ;
#18258=CARTESIAN_POINT ( 'NONE',  ( -110.7369027592740167, -34.07064978273316314, 2.500000000000000000 ) ) ;
#18259=ORIENTED_EDGE ( 'NONE', *, *, #17837, .F. ) ;
#18332=ORIENTED_EDGE ( 'NONE', *, *, #17340, .F. ) ;
#18337=CARTESIAN_POINT ( 'NONE',  ( -128.8620198725179193, 9.173231832019821397, -4.223374618371430245 ) ) ;
#18345=CARTESIAN_POINT ( 'NONE',  ( -126.3445361634317265, 9.599524378652860790, -2.499999999999999112 ) ) ;
#18371=VERTEX_POINT ( 'NONE', #16307 ) ;
#18375=EDGE_CURVE ( 'NONE', #17370, #5722, #13536, .T. ) ;
#18382=ADVANCED_FACE ( 'NONE', ( #16592 ), #17756, .F. ) ;
#18383=CARTESIAN_POINT ( 'NONE',  ( -129.1404785418517918, -15.35070196317932911, -2.500000000000000000 ) ) ;
#18386=DIRECTION ( 'NONE',  ( -1.000000000000000000, 0.000000000000000000, 0.000000000000000000 ) ) ;
#18389=VERTEX_POINT ( 'NONE', #15165 ) ;
#18391=CARTESIAN_POINT ( 'NONE',  ( 0.000000000000000000, 0.000000000000000000, 30.00000000000000000 ) ) ;
#18395=VERTEX_POINT ( 'NONE', #17847 ) ;
#18442=DIRECTION ( 'NONE',  ( 0.000000000000000000, 0.000000000000000000, 1.000000000000000000 ) ) ;
#18454=AXIS2_PLACEMENT_3D ( 'NONE', #16985, #15537, #9848 ) ;
#18467=MECHANICAL_DESIGN_GEOMETRIC_PRESENTATION_REPRESENTATION('',(#12022),#6939);
#18487=ADVANCED_FACE ( 'NONE', ( #14208 ), #970, .F. ) ;
#18494=VECTOR ( 'NONE', #7747, 1000.000000000000000 ) ;
#18519=VECTOR ( 'NONE', #1483, 1000.000000000000000 ) ;
#18520=DIRECTION ( 'NONE',  ( -1.000000000000000000, 0.000000000000000000, 0.000000000000000000 ) ) ;
#18534=DIRECTION ( 'NONE',  ( 1.000000000000000000, 0.000000000000000000, 0.000000000000000000 ) ) ;
#18558=AXIS2_PLACEMENT_3D ( 'NONE', #2405, #10819, #17901 ) ;
#18561=CARTESIAN_POINT ( 'NONE',  ( -94.14047854185179176, 6.938893903907228378E-15, 2.500000000000000000 ) ) ;
#18573=CARTESIAN_POINT ( 'NONE',  ( -129.1237108893556638, -14.52091123662038896, 5.132104245558540612 ) ) ;
#18586=ORIENTED_EDGE ( 'NONE', *, *, #5344, .T. ) ;
#18595=ADVANCED_FACE ( 'NONE', ( #13056, #14314 ), #10031, .F. ) ;
#18601=EDGE_CURVE ( 'NONE', #10401, #5894, #237, .T. ) ;
#18610=ORIENTED_EDGE ( 'NONE', *, *, #2667, .F. ) ;
#18632=ADVANCED_FACE ( 'NONE', ( #4526 ), #5874, .F. ) ;
#18633=EDGE_CURVE ( 'NONE', #17212, #9621, #6924, .T. ) ;
#18647=CYLINDRICAL_SURFACE ( 'NONE', #1772, 20.00000000000001066 ) ;
#18651=CARTESIAN_POINT ( 'NONE',  ( -77.40662104346073136, 32.93835651487657401, 35.00000000000000000 ) ) ;
#18684=DIRECTION ( 'NONE',  ( 0.9868632313631133801, 0.1615579233078773547, -0.000000000000000000 ) ) ;
#18716=DIRECTION ( 'NONE',  ( 0.000000000000000000, 0.000000000000000000, 1.000000000000000000 ) ) ;
#18746=PRODUCT_DEFINITION_FORMATION_WITH_SPECIFIED_SOURCE ( 'ANY', '', #9076, .NOT_KNOWN. ) ;
#18748=ADVANCED_FACE ( 'NONE', ( #7670 ), #1962, .F. ) ;
#18767=ORIENTED_EDGE ( 'NONE', *, *, #14249, .F. ) ;
#18772=AXIS2_PLACEMENT_3D ( 'NONE', #13611, #7473, #14759 ) ;
#18780=EDGE_CURVE ( 'NONE', #16318, #14250, #6628, .T. ) ;
#18781=FACE_OUTER_BOUND ( 'NONE', #15437, .T. ) ;
#18784=DIRECTION ( 'NONE',  ( 3.039628882124824168E-17, 0.000000000000000000, -1.000000000000000000 ) ) ;
ENDSEC;
END-ISO-10303-21;
